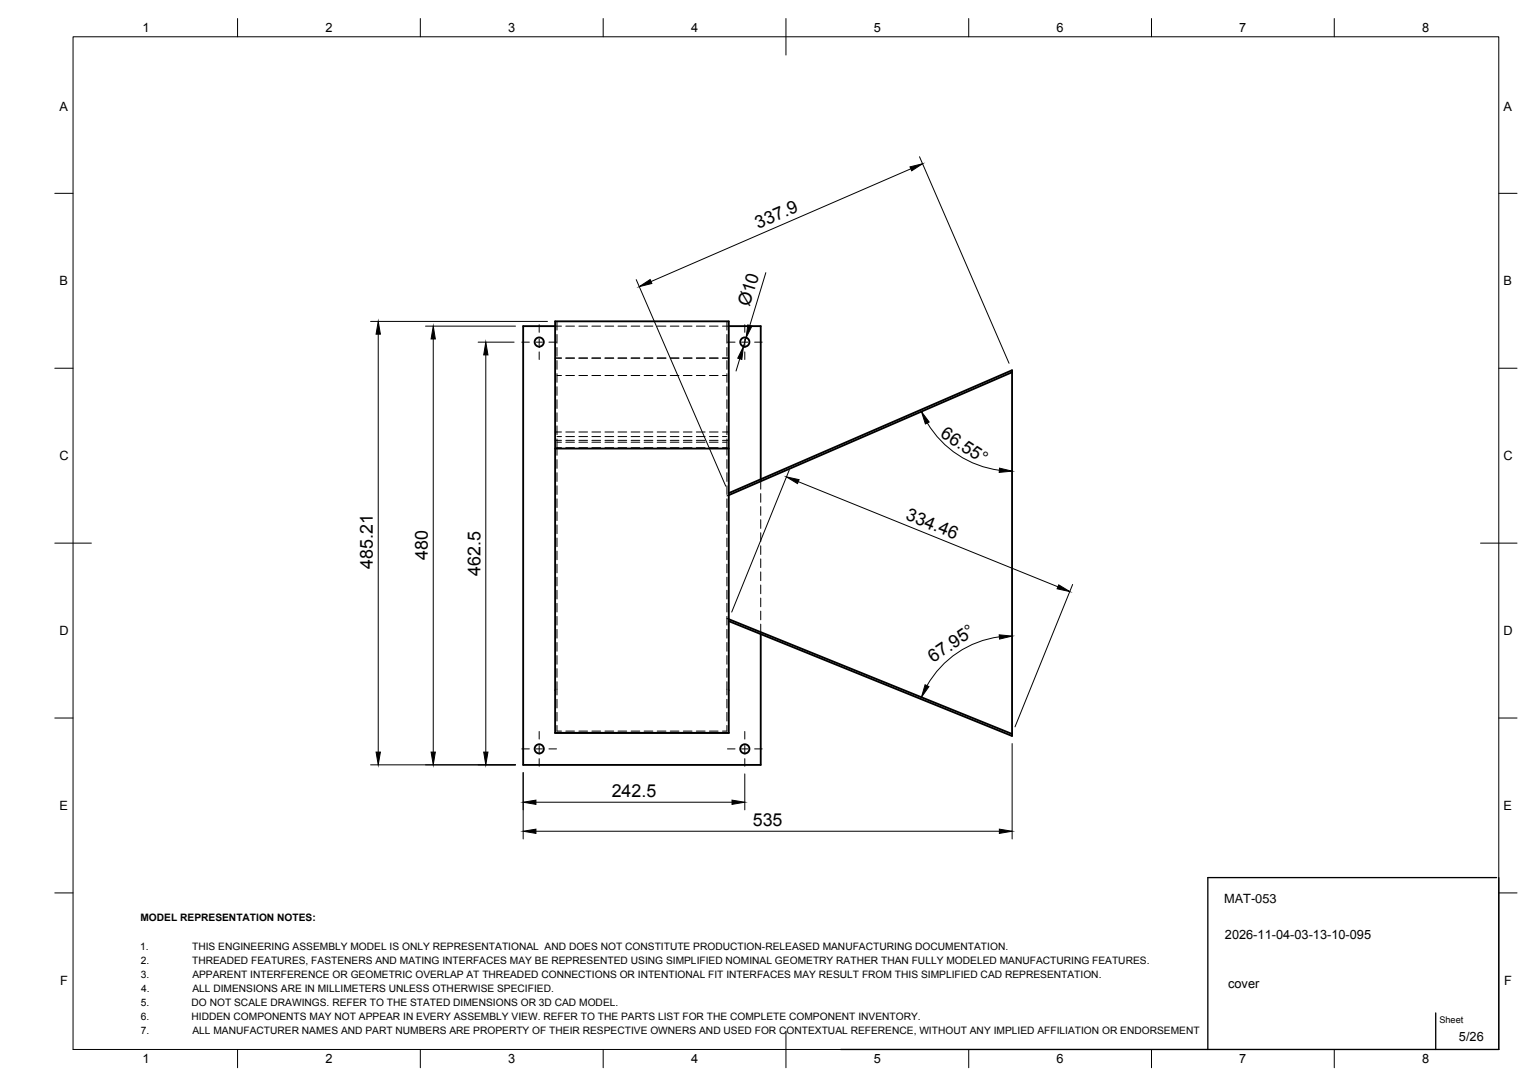
ISO-10303-21;
HEADER;
FILE_DESCRIPTION (('STEP AP214'),
    '1' );
FILE_NAME ('cover.step',
    '2026-10-10T03:43:58',
    ( '' ),
    ( '' ),
    'SwSTEP 2.0',
    'SolidWorks 2026',
    '' );
FILE_SCHEMA (( 'AUTOMOTIVE_DESIGN' ));
ENDSEC;

DATA;
#72=EDGE_CURVE ( 'NONE', #9244, #1149, #61881, .T. ) ;
#95=( NAMED_UNIT ( * ) SI_UNIT ( $, .STERADIAN. ) SOLID_ANGLE_UNIT ( ) );
#152=VECTOR ( 'NONE', #5107, 1000.000000000000000 ) ;
#372=ADVANCED_FACE ( 'NONE', ( #59703 ), #54424, .T. ) ;
#436=ORIENTED_EDGE ( 'NONE', *, *, #28005, .T. ) ;
#560=ORIENTED_EDGE ( 'NONE', *, *, #67855, .T. ) ;
#583=CARTESIAN_POINT ( 'NONE',  ( 544.6745185807129701, 190.0000000000000000, 34.73878747406611467 ) ) ;
#604=LINE ( 'NONE', #43156, #69293 ) ;
#627=EDGE_CURVE ( 'NONE', #45198, #50879, #47422, .T. ) ;
#655=CIRCLE ( 'NONE', #60208, 5.000000000000004441 ) ;
#687=LINE ( 'NONE', #32690, #59969 ) ;
#719=ORIENTED_EDGE ( 'NONE', *, *, #53021, .T. ) ;
#755=EDGE_LOOP ( 'NONE', ( #38002, #54803, #6340, #38216 ) ) ;
#761=AXIS2_PLACEMENT_3D ( 'NONE', #52678, #36171, #19998 ) ;
#765=CYLINDRICAL_SURFACE ( 'NONE', #45215, 498.0000000000000000 ) ;
#855=AXIS2_PLACEMENT_3D ( 'NONE', #17827, #11841, #44185 ) ;
#903=VECTOR ( 'NONE', #22935, 1000.000000000000227 ) ;
#955=ADVANCED_FACE ( 'NONE', ( #29059 ), #50502, .F. ) ;
#967=DIRECTION ( 'NONE',  ( 0.000000000000000000, -1.000000000000000000, 0.000000000000000000 ) ) ;
#1013=FACE_OUTER_BOUND ( 'NONE', #13752, .T. ) ;
#1016=EDGE_CURVE ( 'NONE', #28423, #15873, #49084, .T. ) ;
#1031=LINE ( 'NONE', #55528, #43434 ) ;
#1058=VECTOR ( 'NONE', #1739, 1000.000000000000000 ) ;
#1068=EDGE_LOOP ( 'NONE', ( #54688, #23963, #14484, #64716 ) ) ;
#1072=EDGE_LOOP ( 'NONE', ( #4972, #45772, #7897, #719 ) ) ;
#1100=EDGE_CURVE ( 'NONE', #68856, #49636, #25515, .T. ) ;
#1120=ORIENTED_EDGE ( 'NONE', *, *, #63162, .F. ) ;
#1139=DIRECTION ( 'NONE',  ( -0.000000000000000000, -1.000000000000000000, 0.000000000000000000 ) ) ;
#1149=VERTEX_POINT ( 'NONE', #58195 ) ;
#1267=CARTESIAN_POINT ( 'NONE',  ( 427.4999999999999432, 207.5000000000000284, 20.00000000000000000 ) ) ;
#1301=CARTESIAN_POINT ( 'NONE',  ( 329.1355598199468204, 190.0000000000000000, -129.5087625010780812 ) ) ;
#1353=ORIENTED_EDGE ( 'NONE', *, *, #66788, .F. ) ;
#1368=DIRECTION ( 'NONE',  ( 0.000000000000000000, 0.000000000000000000, -1.000000000000000000 ) ) ;
#1453=DIRECTION ( 'NONE',  ( -1.000000000000000000, -0.000000000000000000, -0.000000000000000000 ) ) ;
#1518=ORIENTED_EDGE ( 'NONE', *, *, #63162, .T. ) ;
#1528=FACE_OUTER_BOUND ( 'NONE', #26038, .T. ) ;
#1554=DIRECTION ( 'NONE',  ( 0.000000000000000000, -1.000000000000000000, 0.000000000000000000 ) ) ;
#1590=ADVANCED_FACE ( 'NONE', ( #39693 ), #61149, .F. ) ;
#1594=VERTEX_POINT ( 'NONE', #29141 ) ;
#1611=DIRECTION ( 'NONE',  ( 0.000000000000000000, 0.000000000000000000, -1.000000000000000000 ) ) ;
#1663=ADVANCED_FACE ( 'NONE', ( #69520, #10102 ), #63570, .F. ) ;
#1722=CARTESIAN_POINT ( 'NONE',  ( -17.50000000000000000, 207.5000000000000284, 0.000000000000000000 ) ) ;
#1724=LINE ( 'NONE', #12275, #14687 ) ;
#1739=DIRECTION ( 'NONE',  ( -1.000000000000000000, -0.000000000000000000, -0.000000000000000000 ) ) ;
#1850=EDGE_CURVE ( 'NONE', #58197, #53112, #45577, .T. ) ;
#1910=CARTESIAN_POINT ( 'NONE',  ( -3.306248862503413655, 500.0000000000000000, -51.64566090791306863 ) ) ;
#1921=PLANE ( 'NONE',  #11654 ) ;
#1944=AXIS2_PLACEMENT_3D ( 'NONE', #14779, #57012, #9163 ) ;
#2001=DIRECTION ( 'NONE',  ( -0.000000000000000000, 0.000000000000000000, 1.000000000000000000 ) ) ;
#2080=DIRECTION ( 'NONE',  ( -1.000000000000000000, 0.000000000000000000, 0.000000000000000000 ) ) ;
#2090=PLANE ( 'NONE',  #24134 ) ;
#2129=DIRECTION ( 'NONE',  ( 0.000000000000000000, 0.000000000000000000, -1.000000000000000000 ) ) ;
#2183=( GEOMETRIC_REPRESENTATION_CONTEXT ( 3 ) GLOBAL_UNCERTAINTY_ASSIGNED_CONTEXT ( ( #2954 ) ) GLOBAL_UNIT_ASSIGNED_CONTEXT ( ( #13188, #10650, #95 ) ) REPRESENTATION_CONTEXT ( 'NONE', 'WORKASPACE' ) );
#2294=VERTEX_POINT ( 'NONE', #16593 ) ;
#2340=CARTESIAN_POINT ( 'NONE',  ( 427.4999999999999432, -17.50000000000000000, 1.999999999999998224 ) ) ;
#2432=FACE_OUTER_BOUND ( 'NONE', #59132, .T. ) ;
#2454=FACE_OUTER_BOUND ( 'NONE', #34954, .T. ) ;
#2458=VECTOR ( 'NONE', #56262, 1000.000000000000000 ) ;
#2459=ORIENTED_EDGE ( 'NONE', *, *, #31851, .T. ) ;
#2461=CARTESIAN_POINT ( 'NONE',  ( -35.00000000000000000, -35.00000000000000000, 2.000000000000000000 ) ) ;
#2510=CARTESIAN_POINT ( 'NONE',  ( 432.4999999999999432, -17.50000000000000000, 1.999999999999998224 ) ) ;
#2542=EDGE_LOOP ( 'NONE', ( #55637, #55611, #67408, #62699 ) ) ;
#2549=CARTESIAN_POINT ( 'NONE',  ( -35.00000000000000000, 225.0000000000000000, 2.000000000000000000 ) ) ;
#2578=LINE ( 'NONE', #60620, #48950 ) ;
#2586=CARTESIAN_POINT ( 'NONE',  ( 124.4094311749753814, 190.0000000000000000, -91.28179539054374914 ) ) ;
#2597=CARTESIAN_POINT ( 'NONE',  ( 422.4999999999999432, -17.50000000000000000, 20.00000000000000000 ) ) ;
#2618=CARTESIAN_POINT ( 'NONE',  ( -12.50000000000000000, -17.50000000000000000, 1.999999999999998224 ) ) ;
#2633=DIRECTION ( 'NONE',  ( 0.000000000000000000, -0.000000000000000000, -1.000000000000000000 ) ) ;
#2634=EDGE_CURVE ( 'NONE', #39735, #19572, #687, .T. ) ;
#2720=LINE ( 'NONE', #3072, #17293 ) ;
#2774=CARTESIAN_POINT ( 'NONE',  ( 444.9999999999999432, 225.0000000000000000, 2.000000000000000000 ) ) ;
#2796=VECTOR ( 'NONE', #29277, 1000.000000000000000 ) ;
#2819=CARTESIAN_POINT ( 'NONE',  ( -35.00000000000000000, -35.00000000000000000, 2.000000000000000000 ) ) ;
#2900=DIRECTION ( 'NONE',  ( -0.000000000000000000, -0.000000000000000000, -1.000000000000000000 ) ) ;
#2931=ORIENTED_EDGE ( 'NONE', *, *, #21135, .T. ) ;
#2932=CARTESIAN_POINT ( 'NONE',  ( -17.50000000000000000, 207.5000000000000284, 20.00000000000000000 ) ) ;
#2954=UNCERTAINTY_MEASURE_WITH_UNIT (LENGTH_MEASURE( 1.000000000000000082E-05 ), #13188, 'distance_accuracy_value', 'NONE');
#2976=DIRECTION ( 'NONE',  ( 0.000000000000000000, -0.000000000000000000, -1.000000000000000000 ) ) ;
#3064=EDGE_CURVE ( 'NONE', #32859, #9244, #55362, .T. ) ;
#3069=EDGE_LOOP ( 'NONE', ( #53736, #43448 ) ) ;
#3072=CARTESIAN_POINT ( 'NONE',  ( -3.306248862503413655, 500.0000000000000000, -91.64566090791306863 ) ) ;
#3079=ORIENTED_EDGE ( 'NONE', *, *, #67167, .T. ) ;
#3080=ORIENTED_EDGE ( 'NONE', *, *, #68526, .T. ) ;
#3126=EDGE_LOOP ( 'NONE', ( #63304, #38150 ) ) ;
#3138=AXIS2_PLACEMENT_3D ( 'NONE', #31491, #3714, #68434 ) ;
#3199=CIRCLE ( 'NONE', #40248, 299.9999999999999432 ) ;
#3206=CARTESIAN_POINT ( 'NONE',  ( 262.2516123306975260, 190.0000000000000000, -21.28179539054375624 ) ) ;
#3323=ORIENTED_EDGE ( 'NONE', *, *, #68445, .F. ) ;
#3328=CARTESIAN_POINT ( 'NONE',  ( 46.68215785206009372, 190.0000000000000000, -77.29788463846088575 ) ) ;
#3448=ORIENTED_EDGE ( 'NONE', *, *, #37030, .T. ) ;
#3462=VERTEX_POINT ( 'NONE', #27498 ) ;
#3473=ORIENTED_EDGE ( 'NONE', *, *, #19374, .F. ) ;
#3528=ORIENTED_EDGE ( 'NONE', *, *, #31290, .F. ) ;
#3596=AXIS2_PLACEMENT_3D ( 'NONE', #19332, #9134, #56272 ) ;
#3663=EDGE_CURVE ( 'NONE', #23198, #50057, #6129, .T. ) ;
#3665=FACE_OUTER_BOUND ( 'NONE', #32196, .T. ) ;
#3714=DIRECTION ( 'NONE',  ( -0.000000000000000000, 0.000000000000000000, 1.000000000000000000 ) ) ;
#3749=CARTESIAN_POINT ( 'NONE',  ( 0.000000000000000000, 190.0000000000000000, 0.000000000000000000 ) ) ;
#3771=VECTOR ( 'NONE', #23467, 1000.000000000000000 ) ;
#3787=VECTOR ( 'NONE', #54739, 1000.000000000000000 ) ;
#3802=CARTESIAN_POINT ( 'NONE',  ( -17.50000000000000000, -17.50000000000000000, 20.00000000000000000 ) ) ;
#3835=ORIENTED_EDGE ( 'NONE', *, *, #21190, .F. ) ;
#3850=CARTESIAN_POINT ( 'NONE',  ( 99.71998884745383407, 0.000000000000000000, 7.478223336038896996 ) ) ;
#3887=DIRECTION ( 'NONE',  ( 0.000000000000000000, -0.000000000000000000, -1.000000000000000000 ) ) ;
#3923=ORIENTED_EDGE ( 'NONE', *, *, #39148, .F. ) ;
#3934=ORIENTED_EDGE ( 'NONE', *, *, #8106, .F. ) ;
#3972=LINE ( 'NONE', #57436, #13122 ) ;
#4135=DIRECTION ( 'NONE',  ( 0.000000000000000000, 1.000000000000000000, -0.000000000000000000 ) ) ;
#4164=DIRECTION ( 'NONE',  ( 0.000000000000000000, -0.000000000000000000, -1.000000000000000000 ) ) ;
#4185=CIRCLE ( 'NONE', #761, 89.99999999999997158 ) ;
#4233=EDGE_CURVE ( 'NONE', #6944, #45198, #13429, .T. ) ;
#4270=AXIS2_PLACEMENT_3D ( 'NONE', #11426, #20963, #48021 ) ;
#4274=EDGE_LOOP ( 'NONE', ( #32274, #55909, #20060, #69556 ) ) ;
#4399=CARTESIAN_POINT ( 'NONE',  ( 544.6745185807129701, 190.0000000000000000, 34.73878747406611467 ) ) ;
#4565=ORIENTED_EDGE ( 'NONE', *, *, #1100, .F. ) ;
#4656=LINE ( 'NONE', #52833, #38629 ) ;
#4697=DIRECTION ( 'NONE',  ( -0.000000000000000000, -0.000000000000000000, -1.000000000000000000 ) ) ;
#4773=ORIENTED_EDGE ( 'NONE', *, *, #26684, .T. ) ;
#4800=EDGE_LOOP ( 'NONE', ( #6610, #17998, #29657, #19956 ) ) ;
#4885=CIRCLE ( 'NONE', #59958, 500.0000000000000000 ) ;
#4916=DIRECTION ( 'NONE',  ( -1.000000000000000000, 0.000000000000000000, 0.000000000000000000 ) ) ;
#4972=ORIENTED_EDGE ( 'NONE', *, *, #28424, .T. ) ;
#4974=CARTESIAN_POINT ( 'NONE',  ( 432.4999999999999432, 207.5000000000000284, 20.00000000000000000 ) ) ;
#5079=AXIS2_PLACEMENT_3D ( 'NONE', #60400, #28035, #12215 ) ;
#5102=DIRECTION ( 'NONE',  ( -1.000000000000000000, 0.000000000000000000, 0.000000000000000000 ) ) ;
#5107=DIRECTION ( 'NONE',  ( 1.000000000000000000, 0.000000000000000000, 0.000000000000000000 ) ) ;
#5231=EDGE_LOOP ( 'NONE', ( #57842, #67743, #13618, #3448 ) ) ;
#5275=DIRECTION ( 'NONE',  ( 0.000000000000000000, 1.000000000000000000, -0.000000000000000000 ) ) ;
#5288=( LENGTH_UNIT ( ) NAMED_UNIT ( * ) SI_UNIT ( .MILLI., .METRE. ) );
#5353=DIRECTION ( 'NONE',  ( -0.000000000000000000, -0.000000000000000000, -1.000000000000000000 ) ) ;
#5418=CIRCLE ( 'NONE', #24575, 299.9999999999999432 ) ;
#5500=ORIENTED_EDGE ( 'NONE', *, *, #38822, .T. ) ;
#5510=DIRECTION ( 'NONE',  ( 0.000000000000000000, -0.000000000000000000, -1.000000000000000000 ) ) ;
#5607=EDGE_CURVE ( 'NONE', #68856, #56615, #2720, .T. ) ;
#5636=CARTESIAN_POINT ( 'NONE',  ( 450.2085304802404266, 0.000000000000000000, -250.0000000000000000 ) ) ;
#5692=PRODUCT_DEFINITION_CONTEXT ( 'detailed design', #47573, 'design' ) ;
#5753=ORIENTED_EDGE ( 'NONE', *, *, #24618, .F. ) ;
#5759=CARTESIAN_POINT ( 'NONE',  ( 311.8713128290285113, 2.000000000000001776, 346.5826552340383842 ) ) ;
#5841=DIRECTION ( 'NONE',  ( 1.000000000000000000, 0.000000000000000000, 0.000000000000000000 ) ) ;
#5867=DIRECTION ( 'NONE',  ( -0.3754025596372949636, 0.9268618657695261165, 0.000000000000000000 ) ) ;
#5916=CIRCLE ( 'NONE', #19450, 97.99999999999994316 ) ;
#5926=LINE ( 'NONE', #38296, #48690 ) ;
#5953=VERTEX_POINT ( 'NONE', #33957 ) ;
#5957=CYLINDRICAL_SURFACE ( 'NONE', #23378, 500.0000000000000000 ) ;
#6094=DIRECTION ( 'NONE',  ( -0.000000000000000000, 0.000000000000000000, -1.000000000000000000 ) ) ;
#6129=LINE ( 'NONE', #64891, #46370 ) ;
#6139=SHAPE_DEFINITION_REPRESENTATION ( #7501, #15003 ) ;
#6221=DIRECTION ( 'NONE',  ( -1.000000000000000000, 0.000000000000000000, 0.000000000000000000 ) ) ;
#6340=ORIENTED_EDGE ( 'NONE', *, *, #27885, .T. ) ;
#6385=CARTESIAN_POINT ( 'NONE',  ( 563.4809901518626702, 2.000000000000001776, 57.79371821540657095 ) ) ;
#6463=PLANE ( 'NONE',  #38849 ) ;
#6504=FACE_OUTER_BOUND ( 'NONE', #40019, .T. ) ;
#6610=ORIENTED_EDGE ( 'NONE', *, *, #41999, .T. ) ;
#6657=LINE ( 'NONE', #22839, #1058 ) ;
#6674=CARTESIAN_POINT ( 'NONE',  ( 410.0000000000000000, 190.0000000000000000, 2.000000000000000000 ) ) ;
#6707=CARTESIAN_POINT ( 'NONE',  ( 46.68215785206009372, 190.0000000000000000, -77.29788463846088575 ) ) ;
#6711=VERTEX_POINT ( 'NONE', #47309 ) ;
#6757=ADVANCED_FACE ( 'NONE', ( #38184 ), #17062, .F. ) ;
#6759=CARTESIAN_POINT ( 'NONE',  ( 563.4809901518626702, 188.0000000000000000, 57.79371821540657095 ) ) ;
#6779=PLANE ( 'NONE',  #31489 ) ;
#6842=CARTESIAN_POINT ( 'NONE',  ( 122.2516123306975402, 190.0000000000000000, -21.28179539054375624 ) ) ;
#6862=ORIENTED_EDGE ( 'NONE', *, *, #67221, .T. ) ;
#6869=CARTESIAN_POINT ( 'NONE',  ( -3.306248862503413655, 500.0000000000000000, -91.64566090791306863 ) ) ;
#6944=VERTEX_POINT ( 'NONE', #68400 ) ;
#6961=ORIENTED_EDGE ( 'NONE', *, *, #32632, .F. ) ;
#7063=DIRECTION ( 'NONE',  ( 0.000000000000000000, 0.000000000000000000, 1.000000000000000000 ) ) ;
#7291=ORIENTED_EDGE ( 'NONE', *, *, #27232, .F. ) ;
#7305=AXIS2_PLACEMENT_3D ( 'NONE', #42807, #17110, #5867 ) ;
#7363=FACE_BOUND ( 'NONE', #15953, .T. ) ;
#7407=EDGE_CURVE ( 'NONE', #8775, #26863, #45567, .T. ) ;
#7420=LINE ( 'NONE', #8453, #39043 ) ;
#7477=PLANE ( 'NONE',  #30552 ) ;
#7487=ORIENTED_EDGE ( 'NONE', *, *, #33804, .T. ) ;
#7501=PRODUCT_DEFINITION_SHAPE ( 'NONE', 'NONE',  #58101 ) ;
#7566=CARTESIAN_POINT ( 'NONE',  ( -17.50000000000000000, -17.50000000000000000, 0.000000000000000000 ) ) ;
#7586=ORIENTED_EDGE ( 'NONE', *, *, #16733, .T. ) ;
#7611=VECTOR ( 'NONE', #14241, 1000.000000000000000 ) ;
#7799=EDGE_CURVE ( 'NONE', #3462, #61751, #2578, .T. ) ;
#7834=AXIS2_PLACEMENT_3D ( 'NONE', #47808, #36233, #21092 ) ;
#7881=ADVANCED_FACE ( 'NONE', ( #1528 ), #6463, .F. ) ;
#7897=ORIENTED_EDGE ( 'NONE', *, *, #23089, .F. ) ;
#7903=DIRECTION ( 'NONE',  ( 0.000000000000000000, 0.000000000000000000, -1.000000000000000000 ) ) ;
#7931=DIRECTION ( 'NONE',  ( -1.000000000000000000, 0.000000000000000000, -0.000000000000000000 ) ) ;
#7940=DIRECTION ( 'NONE',  ( -0.000000000000000000, 0.000000000000000000, 1.000000000000000000 ) ) ;
#7942=ORIENTED_EDGE ( 'NONE', *, *, #68285, .T. ) ;
#7968=LINE ( 'NONE', #18180, #3771 ) ;
#8106=EDGE_CURVE ( 'NONE', #22374, #22712, #21502, .T. ) ;
#8207=VERTEX_POINT ( 'NONE', #25694 ) ;
#8224=DIRECTION ( 'NONE',  ( -0.000000000000000000, -0.000000000000000000, -1.000000000000000000 ) ) ;
#8319=DIRECTION ( 'NONE',  ( 1.000000000000000000, 0.000000000000000000, 0.000000000000000000 ) ) ;
#8380=DIRECTION ( 'NONE',  ( 0.000000000000000000, 0.000000000000000000, -1.000000000000000000 ) ) ;
#8381=CARTESIAN_POINT ( 'NONE',  ( 0.000000000000000000, 190.0000000000000000, 2.000000000000000000 ) ) ;
#8450=AXIS2_PLACEMENT_3D ( 'NONE', #33478, #67813, #23266 ) ;
#8453=CARTESIAN_POINT ( 'NONE',  ( 149.5059104800819796, -64.94516058774519252, -90.98255102680806772 ) ) ;
#8775=VERTEX_POINT ( 'NONE', #2510 ) ;
#8863=VERTEX_POINT ( 'NONE', #23623 ) ;
#8943=SURFACE_STYLE_FILL_AREA ( #57135 ) ;
#9097=EDGE_CURVE ( 'NONE', #27270, #54323, #13093, .T. ) ;
#9121=ORIENTED_EDGE ( 'NONE', *, *, #21343, .F. ) ;
#9134=DIRECTION ( 'NONE',  ( -0.000000000000000000, -1.000000000000000000, 0.000000000000000000 ) ) ;
#9138=EDGE_CURVE ( 'NONE', #33323, #38900, #1031, .T. ) ;
#9163=DIRECTION ( 'NONE',  ( 0.000000000000000000, 0.000000000000000000, -1.000000000000000000 ) ) ;
#9244=VERTEX_POINT ( 'NONE', #2819 ) ;
#9273=AXIS2_PLACEMENT_3D ( 'NONE', #41737, #38090, #32823 ) ;
#9341=FACE_BOUND ( 'NONE', #3126, .T. ) ;
#9414=DIRECTION ( 'NONE',  ( 0.000000000000000000, -1.000000000000000000, 0.000000000000000000 ) ) ;
#9440=FACE_OUTER_BOUND ( 'NONE', #1072, .T. ) ;
#9612=VECTOR ( 'NONE', #27215, 1000.000000000000000 ) ;
#9657=VECTOR ( 'NONE', #33393, 1000.000000000000000 ) ;
#9977=ORIENTED_EDGE ( 'NONE', *, *, #39148, .T. ) ;
#10020=CARTESIAN_POINT ( 'NONE',  ( 410.0000000000000000, 0.000000000000000000, 2.000000000000000000 ) ) ;
#10102=FACE_OUTER_BOUND ( 'NONE', #57610, .T. ) ;
#10125=ORIENTED_EDGE ( 'NONE', *, *, #16907, .T. ) ;
#10159=ORIENTED_EDGE ( 'NONE', *, *, #48623, .F. ) ;
#10170=EDGE_CURVE ( 'NONE', #54229, #41559, #67130, .T. ) ;
#10249=CARTESIAN_POINT ( 'NONE',  ( 262.2516123306975260, 190.0000000000000000, -91.28179539054376335 ) ) ;
#10275=ORIENTED_EDGE ( 'NONE', *, *, #10170, .F. ) ;
#10410=CARTESIAN_POINT ( 'NONE',  ( 0.000000000000000000, -0.2591992991291388049, -2.646296226153046938 ) ) ;
#10519=ORIENTED_EDGE ( 'NONE', *, *, #68285, .F. ) ;
#10650=( NAMED_UNIT ( * ) PLANE_ANGLE_UNIT ( ) SI_UNIT ( $, .RADIAN. ) );
#10773=ORIENTED_EDGE ( 'NONE', *, *, #29862, .T. ) ;
#10921=EDGE_CURVE ( 'NONE', #15873, #38606, #31220, .T. ) ;
#10954=ORIENTED_EDGE ( 'NONE', *, *, #41139, .T. ) ;
#10965=DIRECTION ( 'NONE',  ( 0.000000000000000000, 0.000000000000000000, -1.000000000000000000 ) ) ;
#11077=ORIENTED_EDGE ( 'NONE', *, *, #13353, .T. ) ;
#11182=EDGE_CURVE ( 'NONE', #44112, #5953, #40299, .T. ) ;
#11317=EDGE_CURVE ( 'NONE', #53112, #14479, #18751, .T. ) ;
#11426=CARTESIAN_POINT ( 'NONE',  ( -17.50000000000000000, 207.5000000000000284, 1.999999999999998224 ) ) ;
#11442=ORIENTED_EDGE ( 'NONE', *, *, #63589, .T. ) ;
#11449=( GEOMETRIC_REPRESENTATION_CONTEXT ( 3 ) GLOBAL_UNCERTAINTY_ASSIGNED_CONTEXT ( ( #14872 ) ) GLOBAL_UNIT_ASSIGNED_CONTEXT ( ( #5288, #42902, #58396 ) ) REPRESENTATION_CONTEXT ( 'NONE', 'WORKASPACE' ) );
#11522=CARTESIAN_POINT ( 'NONE',  ( -35.00000000000000000, 225.0000000000000000, 2.000000000000000000 ) ) ;
#11524=EDGE_LOOP ( 'NONE', ( #31151, #7487, #34608, #36208 ) ) ;
#11548=EDGE_CURVE ( 'NONE', #5953, #28478, #3199, .T. ) ;
#11580=VERTEX_POINT ( 'NONE', #21515 ) ;
#11643=VECTOR ( 'NONE', #49675, 1000.000000000000000 ) ;
#11652=DIRECTION ( 'NONE',  ( -0.000000000000000000, -1.000000000000000000, -0.000000000000000000 ) ) ;
#11654=AXIS2_PLACEMENT_3D ( 'NONE', #23374, #44819, #33227 ) ;
#11701=CARTESIAN_POINT ( 'NONE',  ( -35.00000000000000000, 225.0000000000000000, 0.000000000000000000 ) ) ;
#11723=ADVANCED_FACE ( 'NONE', ( #40139 ), #19024, .T. ) ;
#11747=FACE_OUTER_BOUND ( 'NONE', #2542, .T. ) ;
#11770=DIRECTION ( 'NONE',  ( -0.000000000000000000, -1.000000000000000000, -0.000000000000000000 ) ) ;
#11789=ORIENTED_EDGE ( 'NONE', *, *, #4233, .T. ) ;
#11799=ADVANCED_FACE ( 'NONE', ( #22913, #60890 ), #52419, .T. ) ;
#11813=AXIS2_PLACEMENT_3D ( 'NONE', #29215, #42438, #18665 ) ;
#11841=DIRECTION ( 'NONE',  ( 0.000000000000000000, 1.000000000000000000, 0.000000000000000000 ) ) ;
#11878=CARTESIAN_POINT ( 'NONE',  ( 410.0000000000000000, 0.000000000000000000, 2.000000000000000000 ) ) ;
#11926=ADVANCED_FACE ( 'NONE', ( #51728 ), #36243, .F. ) ;
#11952=VERTEX_POINT ( 'NONE', #36593 ) ;
#12022=ORIENTED_EDGE ( 'NONE', *, *, #68445, .T. ) ;
#12032=LINE ( 'NONE', #39126, #903 ) ;
#12055=CARTESIAN_POINT ( 'NONE',  ( 410.0000000000000000, 0.000000000000000000, -90.00000000000000000 ) ) ;
#12148=EDGE_LOOP ( 'NONE', ( #3835, #10275 ) ) ;
#12193=ORIENTED_EDGE ( 'NONE', *, *, #16765, .F. ) ;
#12196=DIRECTION ( 'NONE',  ( 1.000000000000000000, 0.000000000000000000, 0.000000000000000000 ) ) ;
#12203=PLANE ( 'NONE',  #14036 ) ;
#12215=DIRECTION ( 'NONE',  ( 0.000000000000000000, 0.000000000000000000, -1.000000000000000000 ) ) ;
#12275=CARTESIAN_POINT ( 'NONE',  ( 329.1355598199468204, 190.0000000000000000, -129.5087625010780812 ) ) ;
#12361=CARTESIAN_POINT ( 'NONE',  ( 0.000000000000000000, 0.000000000000000000, 2.000000000000000000 ) ) ;
#12363=VECTOR ( 'NONE', #69040, 999.9999999999998863 ) ;
#12429=AXIS2_PLACEMENT_3D ( 'NONE', #47040, #29826, #41426 ) ;
#12549=CARTESIAN_POINT ( 'NONE',  ( 410.0000000000000000, 0.000000000000000000, 0.000000000000000000 ) ) ;
#12624=LINE ( 'NONE', #23874, #55752 ) ;
#12713=EDGE_CURVE ( 'NONE', #22712, #49636, #17250, .T. ) ;
#12777=ORIENTED_EDGE ( 'NONE', *, *, #32544, .F. ) ;
#12905=EDGE_CURVE ( 'NONE', #52426, #26511, #7420, .T. ) ;
#12972=CARTESIAN_POINT ( 'NONE',  ( 563.4809901518626702, 190.0000000000000000, 57.79371821540657095 ) ) ;
#12999=DIRECTION ( 'NONE',  ( 0.000000000000000000, 0.000000000000000000, -1.000000000000000000 ) ) ;
#13016=LINE ( 'NONE', #49929, #20048 ) ;
#13093=CIRCLE ( 'NONE', #20960, 5.000000000000000888 ) ;
#13102=ORIENTED_EDGE ( 'NONE', *, *, #35948, .T. ) ;
#13103=CARTESIAN_POINT ( 'NONE',  ( 311.0133388548732114, 190.0000000000000000, -153.4166086460792826 ) ) ;
#13122=VECTOR ( 'NONE', #19804, 1000.000000000000000 ) ;
#13125=EDGE_CURVE ( 'NONE', #28478, #3462, #24663, .T. ) ;
#13168=EDGE_CURVE ( 'NONE', #34560, #66549, #57932, .T. ) ;
#13183=DIRECTION ( 'NONE',  ( 0.000000000000000000, 0.000000000000000000, -1.000000000000000000 ) ) ;
#13184=DIRECTION ( 'NONE',  ( -0.000000000000000000, -1.000000000000000000, -0.000000000000000000 ) ) ;
#13188=( LENGTH_UNIT ( ) NAMED_UNIT ( * ) SI_UNIT ( .MILLI., .METRE. ) );
#13223=DIRECTION ( 'NONE',  ( 0.000000000000000000, 1.000000000000000000, -0.000000000000000000 ) ) ;
#13245=CARTESIAN_POINT ( 'NONE',  ( 46.68215785206009372, 0.000000000000000000, -77.29788463846088575 ) ) ;
#13340=CARTESIAN_POINT ( 'NONE',  ( 563.4809901518626702, 190.0000000000000000, 57.79371821540657095 ) ) ;
#13353=EDGE_CURVE ( 'NONE', #8863, #25048, #62814, .T. ) ;
#13429=LINE ( 'NONE', #21129, #25103 ) ;
#13468=ORIENTED_EDGE ( 'NONE', *, *, #51660, .T. ) ;
#13476=DIRECTION ( 'NONE',  ( -0.000000000000000000, 0.000000000000000000, 1.000000000000000000 ) ) ;
#13526=CARTESIAN_POINT ( 'NONE',  ( 563.4809901518626702, 190.0000000000000000, 57.79371821540657095 ) ) ;
#13618=ORIENTED_EDGE ( 'NONE', *, *, #45185, .F. ) ;
#13665=ADVANCED_FACE ( 'NONE', ( #57691 ), #14768, .T. ) ;
#13674=CARTESIAN_POINT ( 'NONE',  ( 432.4999999999999432, 207.5000000000000284, 0.000000000000000000 ) ) ;
#13752=EDGE_LOOP ( 'NONE', ( #53113, #24876, #68609, #43593 ) ) ;
#13763=DIRECTION ( 'NONE',  ( -1.000000000000000000, 0.000000000000000000, 0.000000000000000000 ) ) ;
#13773=VECTOR ( 'NONE', #44763, 1000.000000000000000 ) ;
#13804=ORIENTED_EDGE ( 'NONE', *, *, #27232, .T. ) ;
#13820=ADVANCED_FACE ( 'NONE', ( #1013 ), #22114, .T. ) ;
#14009=FACE_OUTER_BOUND ( 'NONE', #755, .T. ) ;
#14021=LINE ( 'NONE', #28823, #23274 ) ;
#14036=AXIS2_PLACEMENT_3D ( 'NONE', #50870, #38944, #49464 ) ;
#14064=CIRCLE ( 'NONE', #8450, 91.99999999999997158 ) ;
#14066=DIRECTION ( 'NONE',  ( -1.000000000000000000, 0.000000000000000000, 0.000000000000000000 ) ) ;
#14069=ADVANCED_FACE ( 'NONE', ( #21338 ), #48744, .T. ) ;
#14074=VECTOR ( 'NONE', #20124, 1000.000000000000000 ) ;
#14241=DIRECTION ( 'NONE',  ( -0.000000000000000000, -0.000000000000000000, -1.000000000000000000 ) ) ;
#14283=PLANE ( 'NONE',  #3138 ) ;
#14349=CARTESIAN_POINT ( 'NONE',  ( -35.00000000000000000, 225.0000000000000000, 2.000000000000000000 ) ) ;
#14368=ORIENTED_EDGE ( 'NONE', *, *, #10921, .T. ) ;
#14392=ORIENTED_EDGE ( 'NONE', *, *, #32938, .T. ) ;
#14449=VERTEX_POINT ( 'NONE', #42029 ) ;
#14479=VERTEX_POINT ( 'NONE', #21949 ) ;
#14484=ORIENTED_EDGE ( 'NONE', *, *, #57557, .T. ) ;
#14687=VECTOR ( 'NONE', #35115, 1000.000000000000000 ) ;
#14706=LINE ( 'NONE', #2774, #68755 ) ;
#14749=VERTEX_POINT ( 'NONE', #18770 ) ;
#14768=PLANE ( 'NONE',  #7834 ) ;
#14779=CARTESIAN_POINT ( 'NONE',  ( 99.71998884745383407, 190.0000000000000000, 7.478223336038896996 ) ) ;
#14858=CARTESIAN_POINT ( 'NONE',  ( 0.000000000000000000, 190.0000000000000000, 2.000000000000000000 ) ) ;
#14872=UNCERTAINTY_MEASURE_WITH_UNIT (LENGTH_MEASURE( 1.000000000000000082E-05 ), #5288, 'distance_accuracy_value', 'NONE');
#14898=ORIENTED_EDGE ( 'NONE', *, *, #58658, .F. ) ;
#14899=ORIENTED_EDGE ( 'NONE', *, *, #67508, .F. ) ;
#15003=SHAPE_REPRESENTATION ( 'cover', ( #66832 ), #17430 ) ;
#15021=ORIENTED_EDGE ( 'NONE', *, *, #7407, .T. ) ;
#15238=CARTESIAN_POINT ( 'NONE',  ( 0.000000000000000000, 0.000000000000000000, 2.000000000000000000 ) ) ;
#15394=DIRECTION ( 'NONE',  ( -0.000000000000000000, -0.000000000000000000, -1.000000000000000000 ) ) ;
#15437=AXIS2_PLACEMENT_3D ( 'NONE', #3850, #41133, #46749 ) ;
#15622=VERTEX_POINT ( 'NONE', #38819 ) ;
#15827=FACE_OUTER_BOUND ( 'NONE', #27928, .T. ) ;
#15828=LINE ( 'NONE', #58723, #40646 ) ;
#15837=AXIS2_PLACEMENT_3D ( 'NONE', #19221, #50895, #46998 ) ;
#15865=DIRECTION ( 'NONE',  ( -0.000000000000000000, -0.000000000000000000, -1.000000000000000000 ) ) ;
#15873=VERTEX_POINT ( 'NONE', #42942 ) ;
#15876=LINE ( 'NONE', #4974, #14074 ) ;
#15953=EDGE_LOOP ( 'NONE', ( #28406, #25946, #47626, #2459 ) ) ;
#15967=DIRECTION ( 'NONE',  ( 1.000000000000000000, 0.000000000000000000, -0.000000000000000000 ) ) ;
#16058=DIRECTION ( 'NONE',  ( 1.000000000000000000, 0.000000000000000000, 0.000000000000000000 ) ) ;
#16153=DIRECTION ( 'NONE',  ( -1.000000000000000000, -0.000000000000000000, -0.000000000000000000 ) ) ;
#16229=CARTESIAN_POINT ( 'NONE',  ( 125.2194818923508848, 188.0000000000000000, 7.478223336038896996 ) ) ;
#16312=CARTESIAN_POINT ( 'NONE',  ( 0.000000000000000000, 190.0000000000000000, 2.000000000000000000 ) ) ;
#16334=ORIENTED_EDGE ( 'NONE', *, *, #21343, .T. ) ;
#16348=CARTESIAN_POINT ( 'NONE',  ( -17.50000000000000000, 207.5000000000000284, 1.999999999999998224 ) ) ;
#16361=VERTEX_POINT ( 'NONE', #2586 ) ;
#16510=FACE_OUTER_BOUND ( 'NONE', #25888, .T. ) ;
#16593=CARTESIAN_POINT ( 'NONE',  ( 432.4999999999999432, -17.50000000000000000, 0.000000000000000000 ) ) ;
#16598=EDGE_CURVE ( 'NONE', #43800, #24193, #60889, .T. ) ;
#16604=CIRCLE ( 'NONE', #4270, 5.000000000000000888 ) ;
#16652=LINE ( 'NONE', #53237, #64671 ) ;
#16733=EDGE_CURVE ( 'NONE', #23556, #19234, #26033, .T. ) ;
#16740=DIRECTION ( 'NONE',  ( -1.000000000000000000, 0.000000000000000000, 0.000000000000000000 ) ) ;
#16752=DIRECTION ( 'NONE',  ( 0.000000000000000000, 0.000000000000000000, -1.000000000000000000 ) ) ;
#16765=EDGE_CURVE ( 'NONE', #52426, #16361, #42872, .T. ) ;
#16805=VECTOR ( 'NONE', #68316, 1000.000000000000000 ) ;
#16870=FILL_AREA_STYLE ('',( #69571 ) ) ;
#16873=ORIENTED_EDGE ( 'NONE', *, *, #19374, .T. ) ;
#16902=EDGE_CURVE ( 'NONE', #18178, #27607, #49897, .T. ) ;
#16907=EDGE_CURVE ( 'NONE', #17378, #28478, #1724, .T. ) ;
#16929=AXIS2_PLACEMENT_3D ( 'NONE', #24746, #55704, #56055 ) ;
#16954=CARTESIAN_POINT ( 'NONE',  ( 311.8713128290285113, 190.0000000000000000, 346.5826552340383842 ) ) ;
#16971=EDGE_LOOP ( 'NONE', ( #34913, #19927, #24153, #42529 ) ) ;
#16994=PLANE ( 'NONE',  #43317 ) ;
#17021=DIRECTION ( 'NONE',  ( -0.000000000000000000, -1.000000000000000000, -0.000000000000000000 ) ) ;
#17062=PLANE ( 'NONE',  #64592 ) ;
#17067=ADVANCED_FACE ( 'NONE', ( #52332 ), #62894, .F. ) ;
#17100=CARTESIAN_POINT ( 'NONE',  ( 329.1355598199467636, 2.000000000000001776, -129.5087625010780812 ) ) ;
#17110=DIRECTION ( 'NONE',  ( 0.9268618657695262275, 0.3754025596372950191, 0.000000000000000000 ) ) ;
#17173=DIRECTION ( 'NONE',  ( 0.000000000000000000, 0.000000000000000000, -1.000000000000000000 ) ) ;
#17206=DIRECTION ( 'NONE',  ( -0.000000000000000000, -1.000000000000000000, -0.000000000000000000 ) ) ;
#17226=CIRCLE ( 'NONE', #65550, 5.000000000000004441 ) ;
#17231=VECTOR ( 'NONE', #54501, 1000.000000000000000 ) ;
#17233=VERTEX_POINT ( 'NONE', #69192 ) ;
#17250=LINE ( 'NONE', #49250, #63738 ) ;
#17293=VECTOR ( 'NONE', #19939, 1000.000000000000000 ) ;
#17327=LINE ( 'NONE', #11701, #11643 ) ;
#17378=VERTEX_POINT ( 'NONE', #61337 ) ;
#17430=( GEOMETRIC_REPRESENTATION_CONTEXT ( 3 ) GLOBAL_UNCERTAINTY_ASSIGNED_CONTEXT ( ( #29000 ) ) GLOBAL_UNIT_ASSIGNED_CONTEXT ( ( #46628, #56851, #51226 ) ) REPRESENTATION_CONTEXT ( 'NONE', 'WORKASPACE' ) );
#17593=PRODUCT_DEFINITION_FORMATION_WITH_SPECIFIED_SOURCE ( 'ANY', '', #45109, .NOT_KNOWN. ) ;
#17597=ORIENTED_EDGE ( 'NONE', *, *, #58189, .F. ) ;
#17667=EDGE_CURVE ( 'NONE', #28478, #25024, #15828, .T. ) ;
#17671=DIRECTION ( 'NONE',  ( -0.000000000000000000, 0.001173758924898823768, 0.9999993111447559313 ) ) ;
#17672=DIRECTION ( 'NONE',  ( 0.000000000000000000, 1.000000000000000000, -0.000000000000000000 ) ) ;
#17688=ORIENTED_EDGE ( 'NONE', *, *, #16902, .F. ) ;
#17708=ORIENTED_EDGE ( 'NONE', *, *, #68531, .F. ) ;
#17737=ORIENTED_EDGE ( 'NONE', *, *, #49048, .F. ) ;
#17747=ORIENTED_EDGE ( 'NONE', *, *, #33006, .F. ) ;
#17827=CARTESIAN_POINT ( 'NONE',  ( -35.00000000000000000, -35.00000000000000000, 2.000000000000000000 ) ) ;
#17870=CARTESIAN_POINT ( 'NONE',  ( 0.000000000000000000, 0.000000000000000000, 2.000000000000000000 ) ) ;
#17933=DIRECTION ( 'NONE',  ( 0.000000000000000000, 0.000000000000000000, -1.000000000000000000 ) ) ;
#17970=ORIENTED_EDGE ( 'NONE', *, *, #59862, .T. ) ;
#17998=ORIENTED_EDGE ( 'NONE', *, *, #72, .F. ) ;
#17999=DIRECTION ( 'NONE',  ( 0.000000000000000000, -0.000000000000000000, -1.000000000000000000 ) ) ;
#18036=MANIFOLD_SOLID_BREP ( 'Cut-Extrude1', #38393 ) ;
#18039=DIRECTION ( 'NONE',  ( 0.000000000000000000, -0.000000000000000000, -1.000000000000000000 ) ) ;
#18053=VECTOR ( 'NONE', #53939, 1000.000000000000000 ) ;
#18147=DIRECTION ( 'NONE',  ( -0.000000000000000000, -0.000000000000000000, -1.000000000000000000 ) ) ;
#18165=VECTOR ( 'NONE', #53831, 1000.000000000000000 ) ;
#18178=VERTEX_POINT ( 'NONE', #6674 ) ;
#18180=CARTESIAN_POINT ( 'NONE',  ( -12.50000000000000000, -17.50000000000000000, 20.00000000000000000 ) ) ;
#18281=CARTESIAN_POINT ( 'NONE',  ( -1.148430018225573557, 500.0000000000000000, -53.65523180892861177 ) ) ;
#18330=PLANE ( 'NONE',  #31153 ) ;
#18365=CARTESIAN_POINT ( 'NONE',  ( 450.2085304802404835, 0.000000000000000000, -219.9999999999999147 ) ) ;
#18402=AXIS2_PLACEMENT_3D ( 'NONE', #59592, #11770, #22328 ) ;
#18447=VECTOR ( 'NONE', #8224, 1000.000000000000000 ) ;
#18452=DIRECTION ( 'NONE',  ( -0.000000000000000000, -1.000000000000000000, 0.000000000000000000 ) ) ;
#18494=ORIENTED_EDGE ( 'NONE', *, *, #43804, .T. ) ;
#18520=ADVANCED_FACE ( 'NONE', ( #62496 ), #67427, .F. ) ;
#18593=DIRECTION ( 'NONE',  ( 0.000000000000000000, 1.000000000000000000, 0.000000000000000000 ) ) ;
#18595=AXIS2_PLACEMENT_3D ( 'NONE', #1722, #28448, #48480 ) ;
#18603=CARTESIAN_POINT ( 'NONE',  ( 0.000000000000000000, 190.0000000000000000, 0.000000000000000000 ) ) ;
#18611=CARTESIAN_POINT ( 'NONE',  ( 0.000000000000000000, 190.0000000000000000, 0.000000000000000000 ) ) ;
#18665=DIRECTION ( 'NONE',  ( 1.000000000000000000, 0.000000000000000000, 0.000000000000000000 ) ) ;
#18750=EDGE_CURVE ( 'NONE', #66549, #23198, #39287, .T. ) ;
#18751=CIRCLE ( 'NONE', #34643, 498.0000000000000000 ) ;
#18770=CARTESIAN_POINT ( 'NONE',  ( 444.9999999999999432, -35.00000000000000000, 2.000000000000000000 ) ) ;
#18944=CIRCLE ( 'NONE', #34720, 5.000000000000004441 ) ;
#18973=LINE ( 'NONE', #40422, #35773 ) ;
#18984=DIRECTION ( 'NONE',  ( -0.000000000000000000, -0.000000000000000000, -1.000000000000000000 ) ) ;
#19000=CYLINDRICAL_SURFACE ( 'NONE', #43736, 5.000000000000000888 ) ;
#19024=PLANE ( 'NONE',  #41354 ) ;
#19066=LINE ( 'NONE', #40520, #63922 ) ;
#19072=AXIS2_PLACEMENT_3D ( 'NONE', #583, #43823, #16752 ) ;
#19158=ORIENTED_EDGE ( 'NONE', *, *, #29375, .F. ) ;
#19221=CARTESIAN_POINT ( 'NONE',  ( 311.8713128290285113, 190.0000000000000000, 346.5826552340383842 ) ) ;
#19234=VERTEX_POINT ( 'NONE', #5636 ) ;
#19254=DIRECTION ( 'NONE',  ( 0.000000000000000000, 0.000000000000000000, -1.000000000000000000 ) ) ;
#19327=LINE ( 'NONE', #23917, #25538 ) ;
#19332=CARTESIAN_POINT ( 'NONE',  ( 563.4809901518626702, 188.0000000000000000, 57.79371821540657095 ) ) ;
#19374=EDGE_CURVE ( 'NONE', #17233, #11580, #36457, .T. ) ;
#19450=AXIS2_PLACEMENT_3D ( 'NONE', #30179, #4135, #8380 ) ;
#19572=VERTEX_POINT ( 'NONE', #43444 ) ;
#19598=AXIS2_PLACEMENT_3D ( 'NONE', #16348, #33238, #37113 ) ;
#19601=AXIS2_PLACEMENT_3D ( 'NONE', #43581, #32353, #37613 ) ;
#19642=LINE ( 'NONE', #18611, #34530 ) ;
#19792=ORIENTED_EDGE ( 'NONE', *, *, #11548, .T. ) ;
#19799=DIRECTION ( 'NONE',  ( -0.000000000000000000, -0.000000000000000000, -1.000000000000000000 ) ) ;
#19804=DIRECTION ( 'NONE',  ( 0.000000000000000000, 0.000000000000000000, -1.000000000000000000 ) ) ;
#19815=EDGE_LOOP ( 'NONE', ( #26290, #49775, #10519, #19869 ) ) ;
#19840=SURFACE_STYLE_USAGE ( .BOTH. , #68040 ) ;
#19846=CARTESIAN_POINT ( 'NONE',  ( 444.9999999999999432, 225.0000000000000000, 0.000000000000000000 ) ) ;
#19852=DIRECTION ( 'NONE',  ( -1.000000000000000000, 0.000000000000000000, 0.000000000000000000 ) ) ;
#19859=ADVANCED_FACE ( 'NONE', ( #44903 ), #12203, .T. ) ;
#19869=ORIENTED_EDGE ( 'NONE', *, *, #62745, .T. ) ;
#19927=ORIENTED_EDGE ( 'NONE', *, *, #48623, .T. ) ;
#19939=DIRECTION ( 'NONE',  ( -1.000000000000000000, -0.000000000000000000, -0.000000000000000000 ) ) ;
#19956=ORIENTED_EDGE ( 'NONE', *, *, #50653, .T. ) ;
#19960=EDGE_LOOP ( 'NONE', ( #16873, #20474, #9121, #42355 ) ) ;
#19998=DIRECTION ( 'NONE',  ( 0.000000000000000000, 0.000000000000000000, -1.000000000000000000 ) ) ;
#20048=VECTOR ( 'NONE', #17933, 1000.000000000000000 ) ;
#20060=ORIENTED_EDGE ( 'NONE', *, *, #25029, .F. ) ;
#20124=DIRECTION ( 'NONE',  ( -0.000000000000000000, -0.000000000000000000, -1.000000000000000000 ) ) ;
#20293=DIRECTION ( 'NONE',  ( -0.000000000000000000, -1.000000000000000000, 0.000000000000000000 ) ) ;
#20317=CARTESIAN_POINT ( 'NONE',  ( 410.0000000000000000, 190.0000000000000000, 0.000000000000000000 ) ) ;
#20463=LINE ( 'NONE', #35272, #46748 ) ;
#20474=ORIENTED_EDGE ( 'NONE', *, *, #36518, .F. ) ;
#20579=FACE_BOUND ( 'NONE', #51834, .T. ) ;
#20644=ADVANCED_FACE ( 'NONE', ( #45390 ), #45743, .F. ) ;
#20732=ORIENTED_EDGE ( 'NONE', *, *, #34405, .T. ) ;
#20840=VECTOR ( 'NONE', #45212, 1000.000000000000000 ) ;
#20960=AXIS2_PLACEMENT_3D ( 'NONE', #43222, #47469, #4916 ) ;
#20963=DIRECTION ( 'NONE',  ( -0.000000000000000000, 0.000000000000000000, 1.000000000000000000 ) ) ;
#20973=ORIENTED_EDGE ( 'NONE', *, *, #5607, .T. ) ;
#20996=ORIENTED_EDGE ( 'NONE', *, *, #1850, .T. ) ;
#21092=DIRECTION ( 'NONE',  ( 0.000000000000000000, -0.9999993111447558203, 0.001173758924898823551 ) ) ;
#21121=CARTESIAN_POINT ( 'NONE',  ( 410.0000000000000000, 190.0000000000000000, 0.000000000000000000 ) ) ;
#21129=CARTESIAN_POINT ( 'NONE',  ( -22.50000000000000355, 207.5000000000000284, 20.00000000000000000 ) ) ;
#21132=SURFACE_SIDE_STYLE ('',( #69306 ) ) ;
#21134=ORIENTED_EDGE ( 'NONE', *, *, #66760, .T. ) ;
#21135=EDGE_CURVE ( 'NONE', #59365, #28423, #5916, .T. ) ;
#21187=DIRECTION ( 'NONE',  ( -0.000000000000000000, -0.000000000000000000, -1.000000000000000000 ) ) ;
#21190=EDGE_CURVE ( 'NONE', #41559, #54229, #47498, .T. ) ;
#21244=ORIENTED_EDGE ( 'NONE', *, *, #16902, .T. ) ;
#21260=DIRECTION ( 'NONE',  ( -0.000000000000000000, -1.000000000000000000, -0.000000000000000000 ) ) ;
#21338=FACE_OUTER_BOUND ( 'NONE', #63270, .T. ) ;
#21340=CARTESIAN_POINT ( 'NONE',  ( 99.71998884745383407, 190.0000000000000000, 7.478223336038896996 ) ) ;
#21343=EDGE_CURVE ( 'NONE', #61832, #28258, #27299, .T. ) ;
#21404=ADVANCED_BREP_SHAPE_REPRESENTATION ( '', ( #65110, #18036, #66832 ), #17430 ) ;
#21502=LINE ( 'NONE', #16229, #45626 ) ;
#21507=LINE ( 'NONE', #26797, #52044 ) ;
#21515=CARTESIAN_POINT ( 'NONE',  ( 410.0000000000000000, 0.000000000000000000, 0.000000000000000000 ) ) ;
#21517=VECTOR ( 'NONE', #29572, 1000.000000000000227 ) ;
#21556=LINE ( 'NONE', #42672, #47852 ) ;
#21615=LINE ( 'NONE', #27938, #56259 ) ;
#21738=ORIENTED_EDGE ( 'NONE', *, *, #46200, .T. ) ;
#21902=EDGE_LOOP ( 'NONE', ( #26574, #45100, #58690, #42968, #31610, #13468, #38650, #35437 ) ) ;
#21949=CARTESIAN_POINT ( 'NONE',  ( 47.74291447196797833, 2.000000000000001776, -75.60236247897087480 ) ) ;
#22114=CYLINDRICAL_SURFACE ( 'NONE', #51668, 91.99999999999997158 ) ;
#22168=CARTESIAN_POINT ( 'NONE',  ( -35.00000000000000000, -35.00000000000000000, 0.000000000000000000 ) ) ;
#22193=AXIS2_PLACEMENT_3D ( 'NONE', #13526, #18452, #13183 ) ;
#22219=FACE_OUTER_BOUND ( 'NONE', #1068, .T. ) ;
#22270=CARTESIAN_POINT ( 'NONE',  ( -35.00000000000000000, 225.0000000000000000, 0.000000000000000000 ) ) ;
#22291=EDGE_LOOP ( 'NONE', ( #17970, #27405, #69147, #22307 ) ) ;
#22307=ORIENTED_EDGE ( 'NONE', *, *, #65368, .T. ) ;
#22328=DIRECTION ( 'NONE',  ( 0.000000000000000000, 0.000000000000000000, -1.000000000000000000 ) ) ;
#22330=EDGE_CURVE ( 'NONE', #26863, #8775, #17226, .T. ) ;
#22373=ORIENTED_EDGE ( 'NONE', *, *, #29287, .T. ) ;
#22374=VERTEX_POINT ( 'NONE', #66716 ) ;
#22463=CARTESIAN_POINT ( 'NONE',  ( 410.0000000000000000, 190.0000000000000000, -90.00000000000000000 ) ) ;
#22474=LINE ( 'NONE', #43913, #9657 ) ;
#22615=ADVANCED_FACE ( 'NONE', ( #11747 ), #1921, .F. ) ;
#22680=DIRECTION ( 'NONE',  ( 0.000000000000000000, 0.000000000000000000, -1.000000000000000000 ) ) ;
#22712=VERTEX_POINT ( 'NONE', #36692 ) ;
#22742=LINE ( 'NONE', #28009, #25147 ) ;
#22839=CARTESIAN_POINT ( 'NONE',  ( 122.2516123306975402, 190.0000000000000000, -91.28179539054376335 ) ) ;
#22881=ORIENTED_EDGE ( 'NONE', *, *, #67167, .F. ) ;
#22913=FACE_BOUND ( 'NONE', #55951, .T. ) ;
#22935=DIRECTION ( 'NONE',  ( 0.3962817440048566620, 0.9137562205704280460, -0.08950055160341972849 ) ) ;
#23089=EDGE_CURVE ( 'NONE', #61986, #32859, #61938, .T. ) ;
#23136=EDGE_CURVE ( 'NONE', #43935, #61832, #66774, .T. ) ;
#23162=VECTOR ( 'NONE', #65313, 1000.000000000000000 ) ;
#23198=VERTEX_POINT ( 'NONE', #21121 ) ;
#23266=DIRECTION ( 'NONE',  ( 0.000000000000000000, 0.000000000000000000, -1.000000000000000000 ) ) ;
#23274=VECTOR ( 'NONE', #66468, 1000.000000000000000 ) ;
#23286=CARTESIAN_POINT ( 'NONE',  ( 0.000000000000000000, 500.0000000000000000, 0.000000000000000000 ) ) ;
#23334=CARTESIAN_POINT ( 'NONE',  ( 324.1677456657756125, 188.0000000000000000, -123.1183350412580779 ) ) ;
#23374=CARTESIAN_POINT ( 'NONE',  ( 0.000000000000000000, -0.1068809833119260672, -91.05865558859387932 ) ) ;
#23378=AXIS2_PLACEMENT_3D ( 'NONE', #65414, #17206, #38679 ) ;
#23384=VECTOR ( 'NONE', #15865, 1000.000000000000000 ) ;
#23418=CIRCLE ( 'NONE', #68351, 5.000000000000000888 ) ;
#23428=EDGE_LOOP ( 'NONE', ( #68713, #25660 ) ) ;
#23457=EDGE_CURVE ( 'NONE', #6944, #38976, #40944, .T. ) ;
#23467=DIRECTION ( 'NONE',  ( -0.000000000000000000, -0.000000000000000000, -1.000000000000000000 ) ) ;
#23556=VERTEX_POINT ( 'NONE', #48210 ) ;
#23595=ORIENTED_EDGE ( 'NONE', *, *, #22330, .F. ) ;
#23618=DIRECTION ( 'NONE',  ( 0.000000000000000000, -0.000000000000000000, 1.000000000000000000 ) ) ;
#23623=CARTESIAN_POINT ( 'NONE',  ( -22.50000000000000355, -17.50000000000000000, 1.999999999999998224 ) ) ;
#23755=CYLINDRICAL_SURFACE ( 'NONE', #31438, 5.000000000000004441 ) ;
#23798=VECTOR ( 'NONE', #52743, 1000.000000000000000 ) ;
#23831=ADVANCED_FACE ( 'NONE', ( #28024 ), #32276, .T. ) ;
#23867=DIRECTION ( 'NONE',  ( -0.000000000000000000, -1.000000000000000000, -0.000000000000000000 ) ) ;
#23874=CARTESIAN_POINT ( 'NONE',  ( 410.0000000000000000, 0.000000000000000000, 2.000000000000000000 ) ) ;
#23875=DIRECTION ( 'NONE',  ( -1.000000000000000000, 0.000000000000000000, 0.000000000000000000 ) ) ;
#23917=CARTESIAN_POINT ( 'NONE',  ( -12.50000000000000000, 207.5000000000000284, 20.00000000000000000 ) ) ;
#23963=ORIENTED_EDGE ( 'NONE', *, *, #27948, .T. ) ;
#23999=ORIENTED_EDGE ( 'NONE', *, *, #61245, .T. ) ;
#24096=DIRECTION ( 'NONE',  ( -1.000000000000000000, 0.000000000000000000, 0.000000000000000000 ) ) ;
#24134=AXIS2_PLACEMENT_3D ( 'NONE', #18603, #28816, #66810 ) ;
#24141=DIRECTION ( 'NONE',  ( -0.000000000000000000, -0.000000000000000000, -1.000000000000000000 ) ) ;
#24153=ORIENTED_EDGE ( 'NONE', *, *, #68245, .T. ) ;
#24193=VERTEX_POINT ( 'NONE', #28649 ) ;
#24254=EDGE_LOOP ( 'NONE', ( #19158, #58420, #25715, #22881, #17747, #12193 ) ) ;
#24321=DIRECTION ( 'NONE',  ( -1.000000000000000000, 0.000000000000000000, 0.000000000000000000 ) ) ;
#24356=LINE ( 'NONE', #34908, #13773 ) ;
#24448=PLANE ( 'NONE',  #63772 ) ;
#24524=ORIENTED_EDGE ( 'NONE', *, *, #62082, .F. ) ;
#24525=FACE_BOUND ( 'NONE', #68964, .T. ) ;
#24575=AXIS2_PLACEMENT_3D ( 'NONE', #6759, #1139, #28208 ) ;
#24618=EDGE_CURVE ( 'NONE', #15622, #44112, #60107, .T. ) ;
#24640=EDGE_CURVE ( 'NONE', #50057, #34560, #33683, .T. ) ;
#24663=CIRCLE ( 'NONE', #63958, 299.9999999999999432 ) ;
#24717=LINE ( 'NONE', #57403, #16805 ) ;
#24746=CARTESIAN_POINT ( 'NONE',  ( 563.4809901518626702, 190.0000000000000000, 57.79371821540657095 ) ) ;
#24785=CARTESIAN_POINT ( 'NONE',  ( 99.71998884745383407, 2.000000000000000000, 7.478223336038896996 ) ) ;
#24847=VECTOR ( 'NONE', #49152, 1000.000000000000000 ) ;
#24859=FACE_OUTER_BOUND ( 'NONE', #4274, .T. ) ;
#24876=ORIENTED_EDGE ( 'NONE', *, *, #31851, .F. ) ;
#24899=ORIENTED_EDGE ( 'NONE', *, *, #45762, .F. ) ;
#24905=FACE_OUTER_BOUND ( 'NONE', #4800, .T. ) ;
#24954=CIRCLE ( 'NONE', #66393, 300.0000000000000000 ) ;
#25024=VERTEX_POINT ( 'NONE', #50461 ) ;
#25029=EDGE_CURVE ( 'NONE', #31022, #55566, #49739, .T. ) ;
#25048=VERTEX_POINT ( 'NONE', #2618 ) ;
#25085=ORIENTED_EDGE ( 'NONE', *, *, #2634, .T. ) ;
#25086=FACE_OUTER_BOUND ( 'NONE', #32574, .T. ) ;
#25103=VECTOR ( 'NONE', #47487, 1000.000000000000000 ) ;
#25147=VECTOR ( 'NONE', #24141, 1000.000000000000000 ) ;
#25269=CARTESIAN_POINT ( 'NONE',  ( 262.2516123306975260, 190.0000000000000000, -91.28179539054376335 ) ) ;
#25331=DIRECTION ( 'NONE',  ( -0.000000000000000000, -0.000000000000000000, -1.000000000000000000 ) ) ;
#25341=AXIS2_PLACEMENT_3D ( 'NONE', #23286, #44731, #17999 ) ;
#25416=CARTESIAN_POINT ( 'NONE',  ( 311.8713128290285113, 188.0000000000000000, -151.4173447659616443 ) ) ;
#25515=LINE ( 'NONE', #35020, #46374 ) ;
#25538=VECTOR ( 'NONE', #18984, 1000.000000000000000 ) ;
#25583=CIRCLE ( 'NONE', #34580, 5.000000000000004441 ) ;
#25660=ORIENTED_EDGE ( 'NONE', *, *, #29287, .F. ) ;
#25694=CARTESIAN_POINT ( 'NONE',  ( 422.4999999999999432, 207.5000000000000284, 0.000000000000000000 ) ) ;
#25715=ORIENTED_EDGE ( 'NONE', *, *, #37030, .F. ) ;
#25759=ORIENTED_EDGE ( 'NONE', *, *, #13168, .F. ) ;
#25844=ORIENTED_EDGE ( 'NONE', *, *, #29862, .F. ) ;
#25888=EDGE_LOOP ( 'NONE', ( #58484, #63953, #22373, #1120 ) ) ;
#25946=ORIENTED_EDGE ( 'NONE', *, *, #1016, .F. ) ;
#26033=LINE ( 'NONE', #57699, #23798 ) ;
#26038=EDGE_LOOP ( 'NONE', ( #47584, #50216, #24524, #3079 ) ) ;
#26043=ORIENTED_EDGE ( 'NONE', *, *, #51492, .T. ) ;
#26048=PLANE ( 'NONE',  #855 ) ;
#26191=EDGE_LOOP ( 'NONE', ( #31822, #43272, #20732, #25085 ) ) ;
#26192=ORIENTED_EDGE ( 'NONE', *, *, #28005, .F. ) ;
#26236=EDGE_CURVE ( 'NONE', #22374, #16361, #21556, .T. ) ;
#26290=ORIENTED_EDGE ( 'NONE', *, *, #25029, .T. ) ;
#26396=DIRECTION ( 'NONE',  ( 0.000000000000000000, 0.000000000000000000, -1.000000000000000000 ) ) ;
#26414=CARTESIAN_POINT ( 'NONE',  ( 0.000000000000000000, 190.0000000000000000, 0.000000000000000000 ) ) ;
#26440=CARTESIAN_POINT ( 'NONE',  ( 99.71998884745383407, 188.0000000000000000, 0.000000000000000000 ) ) ;
#26511=VERTEX_POINT ( 'NONE', #57392 ) ;
#26566=CIRCLE ( 'NONE', #34474, 299.9999999999999432 ) ;
#26574=ORIENTED_EDGE ( 'NONE', *, *, #46200, .F. ) ;
#26580=ORIENTED_EDGE ( 'NONE', *, *, #627, .T. ) ;
#26594=EDGE_CURVE ( 'NONE', #62220, #26511, #67610, .T. ) ;
#26622=EDGE_CURVE ( 'NONE', #54229, #29750, #15876, .T. ) ;
#26684=EDGE_CURVE ( 'NONE', #28328, #6711, #31711, .T. ) ;
#26778=DIRECTION ( 'NONE',  ( -0.3738650651659383151, 0.9230658208099267181, -0.09041240789275073464 ) ) ;
#26797=CARTESIAN_POINT ( 'NONE',  ( -3.306248862503413655, 500.0000000000000000, -91.64566090791306863 ) ) ;
#26863=VERTEX_POINT ( 'NONE', #56994 ) ;
#27035=DIRECTION ( 'NONE',  ( -0.000000000000000000, -1.000000000000000000, 0.000000000000000000 ) ) ;
#27047=VECTOR ( 'NONE', #16153, 1000.000000000000000 ) ;
#27124=VECTOR ( 'NONE', #47441, 1000.000000000000000 ) ;
#27215=DIRECTION ( 'NONE',  ( -0.000000000000000000, -0.000000000000000000, -1.000000000000000000 ) ) ;
#27232=EDGE_CURVE ( 'NONE', #61740, #66549, #31140, .T. ) ;
#27260=EDGE_LOOP ( 'NONE', ( #17708, #51712, #2931, #28767 ) ) ;
#27270=VERTEX_POINT ( 'NONE', #48652 ) ;
#27299=LINE ( 'NONE', #27650, #37411 ) ;
#27401=ORIENTED_EDGE ( 'NONE', *, *, #26594, .T. ) ;
#27405=ORIENTED_EDGE ( 'NONE', *, *, #51492, .F. ) ;
#27498=CARTESIAN_POINT ( 'NONE',  ( 450.2085304802404835, 2.000000000000001776, -219.9999999999999147 ) ) ;
#27537=ADVANCED_FACE ( 'NONE', ( #25086 ), #46523, .F. ) ;
#27602=ORIENTED_EDGE ( 'NONE', *, *, #63589, .F. ) ;
#27607=VERTEX_POINT ( 'NONE', #14858 ) ;
#27650=CARTESIAN_POINT ( 'NONE',  ( 0.000000000000000000, 190.0000000000000000, 0.000000000000000000 ) ) ;
#27876=EDGE_LOOP ( 'NONE', ( #37829, #10159 ) ) ;
#27885=EDGE_CURVE ( 'NONE', #50879, #45198, #42186, .T. ) ;
#27911=DIRECTION ( 'NONE',  ( -0.3754025596372949636, 0.9268618657695261165, 0.000000000000000000 ) ) ;
#27928=EDGE_LOOP ( 'NONE', ( #68295, #57501, #39849, #49530 ) ) ;
#27938=CARTESIAN_POINT ( 'NONE',  ( 410.0000000000000000, 190.0000000000000000, 0.000000000000000000 ) ) ;
#27948=EDGE_CURVE ( 'NONE', #58197, #59365, #66967, .T. ) ;
#28005=EDGE_CURVE ( 'NONE', #65415, #2294, #655, .T. ) ;
#28009=CARTESIAN_POINT ( 'NONE',  ( -22.50000000000000355, -17.50000000000000000, 20.00000000000000000 ) ) ;
#28024=FACE_OUTER_BOUND ( 'NONE', #64026, .T. ) ;
#28029=EDGE_CURVE ( 'NONE', #1594, #60452, #22474, .T. ) ;
#28031=EDGE_LOOP ( 'NONE', ( #50504, #21134, #35510, #3528 ) ) ;
#28035=DIRECTION ( 'NONE',  ( -0.000000000000000000, -1.000000000000000000, 0.000000000000000000 ) ) ;
#28089=ADVANCED_FACE ( 'NONE', ( #14009 ), #50257, .F. ) ;
#28181=CARTESIAN_POINT ( 'NONE',  ( 311.8713128290285113, 190.0000000000000000, 346.5826552340383842 ) ) ;
#28206=PLANE ( 'NONE',  #34430 ) ;
#28208=DIRECTION ( 'NONE',  ( 0.000000000000000000, 0.000000000000000000, -1.000000000000000000 ) ) ;
#28209=CARTESIAN_POINT ( 'NONE',  ( 0.000000000000000000, -0.1068809833119260672, -91.05865558859387932 ) ) ;
#28231=EDGE_CURVE ( 'NONE', #61740, #18178, #12624, .T. ) ;
#28258=VERTEX_POINT ( 'NONE', #20317 ) ;
#28281=CARTESIAN_POINT ( 'NONE',  ( -35.00000000000000000, 225.0000000000000000, 2.000000000000000000 ) ) ;
#28328=VERTEX_POINT ( 'NONE', #25269 ) ;
#28374=LINE ( 'NONE', #1301, #56498 ) ;
#28406=ORIENTED_EDGE ( 'NONE', *, *, #10921, .F. ) ;
#28423=VERTEX_POINT ( 'NONE', #55090 ) ;
#28424=EDGE_CURVE ( 'NONE', #55566, #56923, #33661, .T. ) ;
#28448=DIRECTION ( 'NONE',  ( 0.000000000000000000, 0.000000000000000000, -1.000000000000000000 ) ) ;
#28478=VERTEX_POINT ( 'NONE', #17100 ) ;
#28649=CARTESIAN_POINT ( 'NONE',  ( 396.6937511374966334, 500.0000000000000000, -51.64566090791306863 ) ) ;
#28712=DIRECTION ( 'NONE',  ( -0.000000000000000000, -1.000000000000000000, -0.000000000000000000 ) ) ;
#28767=ORIENTED_EDGE ( 'NONE', *, *, #1016, .T. ) ;
#28773=LINE ( 'NONE', #11522, #24847 ) ;
#28816=DIRECTION ( 'NONE',  ( 0.000000000000000000, 0.000000000000000000, -1.000000000000000000 ) ) ;
#28823=CARTESIAN_POINT ( 'NONE',  ( 450.2085304802404266, 190.0000000000000000, -250.0000000000000000 ) ) ;
#28963=ORIENTED_EDGE ( 'NONE', *, *, #12905, .T. ) ;
#28972=DIRECTION ( 'NONE',  ( -0.000000000000000000, -1.000000000000000000, -0.000000000000000000 ) ) ;
#29000=UNCERTAINTY_MEASURE_WITH_UNIT (LENGTH_MEASURE( 1.000000000000000082E-05 ), #46628, 'distance_accuracy_value', 'NONE');
#29023=FACE_OUTER_BOUND ( 'NONE', #64242, .T. ) ;
#29031=DIRECTION ( 'NONE',  ( -1.048079516971690241E-11, 0.000000000000000000, -1.000000000000000000 ) ) ;
#29048=ORIENTED_EDGE ( 'NONE', *, *, #45762, .T. ) ;
#29059=FACE_OUTER_BOUND ( 'NONE', #52208, .T. ) ;
#29141=CARTESIAN_POINT ( 'NONE',  ( 259.2042601260359334, 188.0000000000000000, -23.09547038499562888 ) ) ;
#29150=CARTESIAN_POINT ( 'NONE',  ( 410.0000000000000000, 190.0000000000000000, 2.000000000000000000 ) ) ;
#29215=CARTESIAN_POINT ( 'NONE',  ( 427.4999999999999432, -17.50000000000000000, 1.999999999999998224 ) ) ;
#29277=DIRECTION ( 'NONE',  ( -0.000000000000000000, -0.000000000000000000, -1.000000000000000000 ) ) ;
#29287=EDGE_CURVE ( 'NONE', #29750, #8207, #58058, .T. ) ;
#29375=EDGE_CURVE ( 'NONE', #28328, #52426, #604, .T. ) ;
#29555=AXIS2_PLACEMENT_3D ( 'NONE', #12972, #23867, #45310 ) ;
#29572=DIRECTION ( 'NONE',  ( 0.3962817440048567175, 0.9137562205704280460, -0.08950055160341974236 ) ) ;
#29638=EDGE_CURVE ( 'NONE', #38509, #23556, #14021, .T. ) ;
#29657=ORIENTED_EDGE ( 'NONE', *, *, #3064, .F. ) ;
#29696=PLANE ( 'NONE',  #45715 ) ;
#29708=ADVANCED_FACE ( 'NONE', ( #2432 ), #50614, .T. ) ;
#29712=EDGE_CURVE ( 'NONE', #61832, #17233, #19642, .T. ) ;
#29750=VERTEX_POINT ( 'NONE', #13674 ) ;
#29754=LINE ( 'NONE', #69368, #64486 ) ;
#29784=FACE_BOUND ( 'NONE', #3069, .T. ) ;
#29824=DIRECTION ( 'NONE',  ( 1.000000000000000000, 0.000000000000000000, 0.000000000000000000 ) ) ;
#29826=DIRECTION ( 'NONE',  ( 0.000000000000000000, 1.000000000000000000, -0.000000000000000000 ) ) ;
#29862=EDGE_CURVE ( 'NONE', #28258, #30681, #4185, .T. ) ;
#29996=ADVANCED_FACE ( 'NONE', ( #9440 ), #57630, .F. ) ;
#30053=FACE_OUTER_BOUND ( 'NONE', #65926, .T. ) ;
#30179=CARTESIAN_POINT ( 'NONE',  ( 99.71998884745383407, 188.0000000000000000, 7.478223336038896996 ) ) ;
#30337=EDGE_CURVE ( 'NONE', #8207, #29750, #25583, .T. ) ;
#30422=ORIENTED_EDGE ( 'NONE', *, *, #40565, .T. ) ;
#30425=DIRECTION ( 'NONE',  ( -0.000000000000000000, 0.000000000000000000, 1.000000000000000000 ) ) ;
#30477=DIRECTION ( 'NONE',  ( -0.000000000000000000, 0.000000000000000000, 1.000000000000000000 ) ) ;
#30552=AXIS2_PLACEMENT_3D ( 'NONE', #28209, #17671, #66228 ) ;
#30638=VERTEX_POINT ( 'NONE', #65064 ) ;
#30639=CARTESIAN_POINT ( 'NONE',  ( 427.4999999999999432, 207.5000000000000284, 0.000000000000000000 ) ) ;
#30681=VERTEX_POINT ( 'NONE', #39726 ) ;
#30722=ADVANCED_FACE ( 'NONE', ( #43934 ), #5957, .T. ) ;
#30753=CARTESIAN_POINT ( 'NONE',  ( 427.4999999999999432, -17.50000000000000000, 20.00000000000000000 ) ) ;
#30864=DIRECTION ( 'NONE',  ( 1.000000000000000000, 0.000000000000000000, 0.000000000000000000 ) ) ;
#30896=DIRECTION ( 'NONE',  ( 0.000000000000000000, -1.000000000000000000, 0.000000000000000000 ) ) ;
#31022=VERTEX_POINT ( 'NONE', #57209 ) ;
#31140=LINE ( 'NONE', #10020, #9612 ) ;
#31151=ORIENTED_EDGE ( 'NONE', *, *, #22330, .T. ) ;
#31153=AXIS2_PLACEMENT_3D ( 'NONE', #45765, #24321, #39791 ) ;
#31220=LINE ( 'NONE', #52651, #32308 ) ;
#31290=EDGE_CURVE ( 'NONE', #30681, #38509, #52525, .T. ) ;
#31312=ORIENTED_EDGE ( 'NONE', *, *, #68526, .F. ) ;
#31323=ORIENTED_EDGE ( 'NONE', *, *, #23136, .T. ) ;
#31438=AXIS2_PLACEMENT_3D ( 'NONE', #61723, #60687, #55765 ) ;
#31489=AXIS2_PLACEMENT_3D ( 'NONE', #45105, #34221, #18039 ) ;
#31491=CARTESIAN_POINT ( 'NONE',  ( 0.000000000000000000, 0.000000000000000000, 2.000000000000000000 ) ) ;
#31610=ORIENTED_EDGE ( 'NONE', *, *, #29638, .F. ) ;
#31696=EDGE_CURVE ( 'NONE', #43800, #28328, #13016, .T. ) ;
#31708=LINE ( 'NONE', #26440, #50086 ) ;
#31711=LINE ( 'NONE', #10249, #32041 ) ;
#31764=VECTOR ( 'NONE', #65285, 1000.000000000000000 ) ;
#31779=CYLINDRICAL_SURFACE ( 'NONE', #59189, 5.000000000000004441 ) ;
#31822=ORIENTED_EDGE ( 'NONE', *, *, #35435, .F. ) ;
#31851=EDGE_CURVE ( 'NONE', #15622, #38606, #18973, .T. ) ;
#31933=DIRECTION ( 'NONE',  ( 0.000000000000000000, 0.000000000000000000, -1.000000000000000000 ) ) ;
#31944=DIRECTION ( 'NONE',  ( -0.000000000000000000, 0.000000000000000000, 1.000000000000000000 ) ) ;
#32041=VECTOR ( 'NONE', #63031, 1000.000000000000000 ) ;
#32080=DIRECTION ( 'NONE',  ( 0.000000000000000000, 0.000000000000000000, -1.000000000000000000 ) ) ;
#32085=CARTESIAN_POINT ( 'NONE',  ( 450.2085304802404266, 188.0000000000000000, 7.478223336038896996 ) ) ;
#32196=EDGE_LOOP ( 'NONE', ( #41412, #14368, #18494, #19792, #48066, #21738, #62188, #62840, #49779 ) ) ;
#32220=DIRECTION ( 'NONE',  ( -1.048079516971690241E-11, 0.000000000000000000, -1.000000000000000000 ) ) ;
#32240=CARTESIAN_POINT ( 'NONE',  ( 0.000000000000000000, 0.000000000000000000, 0.000000000000000000 ) ) ;
#32274=ORIENTED_EDGE ( 'NONE', *, *, #41999, .F. ) ;
#32276=PLANE ( 'NONE',  #7305 ) ;
#32308=VECTOR ( 'NONE', #68163, 1000.000000000000000 ) ;
#32341=ORIENTED_EDGE ( 'NONE', *, *, #11548, .F. ) ;
#32353=DIRECTION ( 'NONE',  ( -0.000000000000000000, -0.000000000000000000, -1.000000000000000000 ) ) ;
#32389=ORIENTED_EDGE ( 'NONE', *, *, #12905, .F. ) ;
#32449=CARTESIAN_POINT ( 'NONE',  ( 422.4999999999999432, 207.5000000000000284, 1.999999999999998224 ) ) ;
#32467=DIRECTION ( 'NONE',  ( -0.3754023374827052950, 0.9268613172740186590, -0.001087912492708085609 ) ) ;
#32540=EDGE_LOOP ( 'NONE', ( #32832, #7291, #46023, #3080 ) ) ;
#32544=EDGE_CURVE ( 'NONE', #2294, #65415, #18944, .T. ) ;
#32559=CARTESIAN_POINT ( 'NONE',  ( 311.8713128290285113, 188.0000000000000000, 346.5826552340383842 ) ) ;
#32574=EDGE_LOOP ( 'NONE', ( #48315, #46174, #11789, #26580 ) ) ;
#32632=EDGE_CURVE ( 'NONE', #19572, #53112, #54924, .T. ) ;
#32690=CARTESIAN_POINT ( 'NONE',  ( 311.9732115134679020, 188.0000000000000000, -151.4173343409194672 ) ) ;
#32823=DIRECTION ( 'NONE',  ( -1.000000000000000000, 0.000000000000000000, 0.000000000000000000 ) ) ;
#32832=ORIENTED_EDGE ( 'NONE', *, *, #18750, .F. ) ;
#32852=AXIS2_PLACEMENT_3D ( 'NONE', #44701, #33799, #7063 ) ;
#32859=VERTEX_POINT ( 'NONE', #2549 ) ;
#32938=EDGE_CURVE ( 'NONE', #27607, #50057, #19066, .T. ) ;
#32958=VECTOR ( 'NONE', #48450, 1000.000000000000000 ) ;
#33001=EDGE_LOOP ( 'NONE', ( #46038, #62130, #29048, #44251 ) ) ;
#33006=EDGE_CURVE ( 'NONE', #16361, #30638, #6657, .T. ) ;
#33227=DIRECTION ( 'NONE',  ( 0.000000000000000000, -0.9999993111447558203, 0.001173758924898823551 ) ) ;
#33238=DIRECTION ( 'NONE',  ( -0.000000000000000000, 0.000000000000000000, 1.000000000000000000 ) ) ;
#33310=CARTESIAN_POINT ( 'NONE',  ( 444.9999999999999432, -35.00000000000000000, 2.000000000000000000 ) ) ;
#33323=VERTEX_POINT ( 'NONE', #56490 ) ;
#33353=ADVANCED_FACE ( 'NONE', ( #40278 ), #23755, .F. ) ;
#33365=LINE ( 'NONE', #49863, #46408 ) ;
#33386=CARTESIAN_POINT ( 'NONE',  ( 260.0716287634991204, 189.9999999999999432, -91.28179539054374914 ) ) ;
#33393=DIRECTION ( 'NONE',  ( 0.000000000000000000, 0.000000000000000000, -1.000000000000000000 ) ) ;
#33478=CARTESIAN_POINT ( 'NONE',  ( 410.0000000000000000, 2.000000000000001776, -90.00000000000000000 ) ) ;
#33593=EDGE_LOOP ( 'NONE', ( #39521, #63928, #65761, #60754, #34653, #40843, #17737, #5753, #17597 ) ) ;
#33640=CARTESIAN_POINT ( 'NONE',  ( 2.005731055991735623, 188.0000000000000000, 0.000000000000000000 ) ) ;
#33647=VECTOR ( 'NONE', #30864, 1000.000000000000000 ) ;
#33661=LINE ( 'NONE', #38222, #23162 ) ;
#33683=LINE ( 'NONE', #37549, #36530 ) ;
#33751=ORIENTED_EDGE ( 'NONE', *, *, #26684, .F. ) ;
#33799=DIRECTION ( 'NONE',  ( -1.000000000000000000, 0.000000000000000000, 0.000000000000000000 ) ) ;
#33804=EDGE_CURVE ( 'NONE', #8775, #2294, #24717, .T. ) ;
#33957=CARTESIAN_POINT ( 'NONE',  ( 324.1677456657756125, 2.000000000000000000, -123.1183350412580779 ) ) ;
#34078=ORIENTED_EDGE ( 'NONE', *, *, #31696, .T. ) ;
#34107=ORIENTED_EDGE ( 'NONE', *, *, #58658, .T. ) ;
#34145=ADVANCED_FACE ( 'NONE', ( #34845 ), #19000, .F. ) ;
#34221=DIRECTION ( 'NONE',  ( 0.000000000000000000, -1.000000000000000000, 0.000000000000000000 ) ) ;
#34285=CIRCLE ( 'NONE', #54481, 498.0000000000000000 ) ;
#34290=CYLINDRICAL_SURFACE ( 'NONE', #18402, 89.99999999999997158 ) ;
#34315=LINE ( 'NONE', #39924, #7611 ) ;
#34326=VECTOR ( 'NONE', #40253, 1000.000000000000000 ) ;
#34405=EDGE_CURVE ( 'NONE', #33323, #39735, #41503, .T. ) ;
#34430=AXIS2_PLACEMENT_3D ( 'NONE', #51331, #62213, #54226 ) ;
#34474=AXIS2_PLACEMENT_3D ( 'NONE', #64683, #27035, #52732 ) ;
#34530=VECTOR ( 'NONE', #61850, 1000.000000000000000 ) ;
#34560=VERTEX_POINT ( 'NONE', #32240 ) ;
#34580=AXIS2_PLACEMENT_3D ( 'NONE', #30639, #35572, #13763 ) ;
#34608=ORIENTED_EDGE ( 'NONE', *, *, #32544, .T. ) ;
#34643=AXIS2_PLACEMENT_3D ( 'NONE', #5759, #64165, #65212 ) ;
#34653=ORIENTED_EDGE ( 'NONE', *, *, #68543, .F. ) ;
#34720=AXIS2_PLACEMENT_3D ( 'NONE', #62411, #35689, #24096 ) ;
#34798=DIRECTION ( 'NONE',  ( 0.000000000000000000, 1.000000000000000000, -0.000000000000000000 ) ) ;
#34809=CARTESIAN_POINT ( 'NONE',  ( 173.0237957311180708, 69.97204739562489806, -91.14091141288837150 ) ) ;
#34845=FACE_OUTER_BOUND ( 'NONE', #16971, .T. ) ;
#34870=FACE_OUTER_BOUND ( 'NONE', #21902, .T. ) ;
#34885=AXIS2_PLACEMENT_3D ( 'NONE', #4399, #21260, #58881 ) ;
#34908=CARTESIAN_POINT ( 'NONE',  ( 396.6937511374966334, 500.0000000000000000, -51.64566090791306863 ) ) ;
#34913=ORIENTED_EDGE ( 'NONE', *, *, #41139, .F. ) ;
#34946=DIRECTION ( 'NONE',  ( -1.000000000000000000, 0.000000000000000000, 0.000000000000000000 ) ) ;
#34954=EDGE_LOOP ( 'NONE', ( #4773, #43606, #61868, #34078 ) ) ;
#34955=ORIENTED_EDGE ( 'NONE', *, *, #24640, .T. ) ;
#34957=LINE ( 'NONE', #2597, #18447 ) ;
#35020=CARTESIAN_POINT ( 'NONE',  ( -1.148430018225575555, 500.0000000000000000, -0.000000000000000000 ) ) ;
#35028=VECTOR ( 'NONE', #57227, 1000.000000000000000 ) ;
#35115=DIRECTION ( 'NONE',  ( -0.000000000000000000, -1.000000000000000000, -0.000000000000000000 ) ) ;
#35138=AXIS2_PLACEMENT_3D ( 'NONE', #1267, #18147, #16740 ) ;
#35239=LINE ( 'NONE', #13103, #42678 ) ;
#35272=CARTESIAN_POINT ( 'NONE',  ( 122.2516123306975402, 190.0000000000000000, -21.28179539054375624 ) ) ;
#35277=AXIS2_PLACEMENT_3D ( 'NONE', #12055, #49320, #38797 ) ;
#35339=CARTESIAN_POINT ( 'NONE',  ( 122.2516123306975402, 190.0000000000000000, -91.28179539054376335 ) ) ;
#35435=EDGE_CURVE ( 'NONE', #38900, #19572, #42736, .T. ) ;
#35437=ORIENTED_EDGE ( 'NONE', *, *, #9138, .T. ) ;
#35481=DIRECTION ( 'NONE',  ( -0.000000000000000000, -1.000000000000000000, -0.000000000000000000 ) ) ;
#35510=ORIENTED_EDGE ( 'NONE', *, *, #51660, .F. ) ;
#35572=DIRECTION ( 'NONE',  ( 0.000000000000000000, 0.000000000000000000, -1.000000000000000000 ) ) ;
#35626=AXIS2_PLACEMENT_3D ( 'NONE', #41519, #52071, #3887 ) ;
#35682=FILL_AREA_STYLE_COLOUR ( '', #51633 ) ;
#35689=DIRECTION ( 'NONE',  ( 0.000000000000000000, 0.000000000000000000, -1.000000000000000000 ) ) ;
#35773=VECTOR ( 'NONE', #61867, 1000.000000000000000 ) ;
#35780=ADVANCED_FACE ( 'NONE', ( #58533 ), #46962, .F. ) ;
#35804=DIRECTION ( 'NONE',  ( 1.000000000000000000, 0.000000000000000000, -0.000000000000000000 ) ) ;
#35828=CARTESIAN_POINT ( 'NONE',  ( 311.8713128290285113, 2.000000000000001776, -151.4173447659616443 ) ) ;
#35865=CARTESIAN_POINT ( 'NONE',  ( 544.6745185807129701, 0.000000000000000000, 34.73878747406611467 ) ) ;
#35896=APPLICATION_CONTEXT ( 'automotive_design' ) ;
#35948=EDGE_CURVE ( 'NONE', #11952, #24193, #54994, .T. ) ;
#36163=ADVANCED_FACE ( 'NONE', ( #56395 ), #62371, .F. ) ;
#36171=DIRECTION ( 'NONE',  ( -0.000000000000000000, -1.000000000000000000, 0.000000000000000000 ) ) ;
#36198=CLOSED_SHELL ( 'NONE', ( #18520, #69221, #1590, #46587, #59694, #22615, #61380, #54613, #36163, #14069, #30722, #1663, #61453, #38163, #6757, #37707, #7881, #29708, #13665, #11926, #13820, #35780, #52871, #11799, #50385, #60735, #19859, #23831 ) ) ;
#36208=ORIENTED_EDGE ( 'NONE', *, *, #40565, .F. ) ;
#36233=DIRECTION ( 'NONE',  ( -0.000000000000000000, 0.001173758924898823768, 0.9999993111447559313 ) ) ;
#36243=CYLINDRICAL_SURFACE ( 'NONE', #1944, 97.99999999999994316 ) ;
#36359=EDGE_LOOP ( 'NONE', ( #26192, #12777 ) ) ;
#36457=LINE ( 'NONE', #45633, #35028 ) ;
#36518=EDGE_CURVE ( 'NONE', #28258, #11580, #21615, .T. ) ;
#36530=VECTOR ( 'NONE', #967, 1000.000000000000000 ) ;
#36593=CARTESIAN_POINT ( 'NONE',  ( -3.306248862503413655, 500.0000000000000000, -51.64566090791306863 ) ) ;
#36606=CARTESIAN_POINT ( 'NONE',  ( 99.71998884745383407, 190.0000000000000000, 7.478223336038896996 ) ) ;
#36618=ORIENTED_EDGE ( 'NONE', *, *, #33804, .F. ) ;
#36692=CARTESIAN_POINT ( 'NONE',  ( 125.2194818923508848, 188.0000000000000000, -23.09547038499562888 ) ) ;
#36728=AXIS2_PLACEMENT_3D ( 'NONE', #61361, #13184, #7903 ) ;
#36776=FACE_OUTER_BOUND ( 'NONE', #42215, .T. ) ;
#37030=EDGE_CURVE ( 'NONE', #37226, #43800, #69468, .T. ) ;
#37107=FACE_BOUND ( 'NONE', #39399, .T. ) ;
#37113=DIRECTION ( 'NONE',  ( 1.000000000000000000, 0.000000000000000000, 0.000000000000000000 ) ) ;
#37205=ORIENTED_EDGE ( 'NONE', *, *, #41055, .F. ) ;
#37226=VERTEX_POINT ( 'NONE', #6842 ) ;
#37295=ORIENTED_EDGE ( 'NONE', *, *, #3663, .F. ) ;
#37304=ORIENTED_EDGE ( 'NONE', *, *, #68245, .F. ) ;
#37342=DIRECTION ( 'NONE',  ( -0.000000000000000000, -1.000000000000000000, 0.000000000000000000 ) ) ;
#37346=CARTESIAN_POINT ( 'NONE',  ( 99.71998884745383407, 2.000000000000001776, 7.478223336038896996 ) ) ;
#37411=VECTOR ( 'NONE', #16058, 1000.000000000000000 ) ;
#37549=CARTESIAN_POINT ( 'NONE',  ( 0.000000000000000000, 190.0000000000000000, 0.000000000000000000 ) ) ;
#37613=DIRECTION ( 'NONE',  ( -1.000000000000000000, 0.000000000000000000, 0.000000000000000000 ) ) ;
#37657=AXIS2_PLACEMENT_3D ( 'NONE', #44647, #34798, #56236 ) ;
#37707=ADVANCED_FACE ( 'NONE', ( #50378 ), #7477, .F. ) ;
#37759=CIRCLE ( 'NONE', #67076, 5.000000000000000888 ) ;
#37829=ORIENTED_EDGE ( 'NONE', *, *, #13353, .F. ) ;
#37956=DIRECTION ( 'NONE',  ( -1.000000000000000000, 0.000000000000000000, 0.000000000000000000 ) ) ;
#38002=ORIENTED_EDGE ( 'NONE', *, *, #23457, .T. ) ;
#38039=ORIENTED_EDGE ( 'NONE', *, *, #3663, .T. ) ;
#38090=DIRECTION ( 'NONE',  ( 0.000000000000000000, 0.000000000000000000, -1.000000000000000000 ) ) ;
#38150=ORIENTED_EDGE ( 'NONE', *, *, #50125, .F. ) ;
#38163=ADVANCED_FACE ( 'NONE', ( #2454 ), #45003, .F. ) ;
#38184=FACE_OUTER_BOUND ( 'NONE', #5231, .T. ) ;
#38216=ORIENTED_EDGE ( 'NONE', *, *, #4233, .F. ) ;
#38222=CARTESIAN_POINT ( 'NONE',  ( 444.9999999999999432, 225.0000000000000000, 0.000000000000000000 ) ) ;
#38240=CARTESIAN_POINT ( 'NONE',  ( 432.4999999999999432, 207.5000000000000284, 1.999999999999998224 ) ) ;
#38273=MECHANICAL_DESIGN_GEOMETRIC_PRESENTATION_REPRESENTATION('',(#65357),#11449);
#38296=CARTESIAN_POINT ( 'NONE',  ( -3.306248862503413655, 500.0000000000000000, -51.64566090791306863 ) ) ;
#38359=CARTESIAN_POINT ( 'NONE',  ( 311.0133388548732114, 190.0000000000000000, -153.4166086460792826 ) ) ;
#38382=COLOUR_RGB ( '',0.7921568627450980005, 0.8196078431372548767, 0.9333333333333333481 ) ;
#38393=CLOSED_SHELL ( 'NONE', ( #69037, #28089, #17067, #62092, #47733, #64765, #43846, #47620, #20644, #29996, #44953, #11723, #372, #66413, #33353, #34145, #27537, #955 ) ) ;
#38509=VERTEX_POINT ( 'NONE', #45272 ) ;
#38566=LINE ( 'NONE', #33310, #3787 ) ;
#38606=VERTEX_POINT ( 'NONE', #62503 ) ;
#38629=VECTOR ( 'NONE', #5353, 1000.000000000000000 ) ;
#38650=ORIENTED_EDGE ( 'NONE', *, *, #68543, .T. ) ;
#38679=DIRECTION ( 'NONE',  ( 0.000000000000000000, 0.000000000000000000, -1.000000000000000000 ) ) ;
#38797=DIRECTION ( 'NONE',  ( 0.000000000000000000, 0.000000000000000000, -1.000000000000000000 ) ) ;
#38819=CARTESIAN_POINT ( 'NONE',  ( 390.9212159716611836, 188.0000000000000000, 0.000000000000000000 ) ) ;
#38822=EDGE_CURVE ( 'NONE', #24193, #6711, #24356, .T. ) ;
#38849=AXIS2_PLACEMENT_3D ( 'NONE', #49697, #65923, #27911 ) ;
#38900=VERTEX_POINT ( 'NONE', #56346 ) ;
#38931=VECTOR ( 'NONE', #9414, 1000.000000000000000 ) ;
#38944=DIRECTION ( 'NONE',  ( 0.000000000000000000, -0.09748146057682104126, -0.9952373409613456401 ) ) ;
#38976=VERTEX_POINT ( 'NONE', #57053 ) ;
#39043=VECTOR ( 'NONE', #56282, 999.9999999999998863 ) ;
#39126=CARTESIAN_POINT ( 'NONE',  ( 149.6041652118227603, -64.71860240360767591, 1.657799476683943007 ) ) ;
#39148=EDGE_CURVE ( 'NONE', #49636, #62220, #43471, .T. ) ;
#39287=LINE ( 'NONE', #12549, #53317 ) ;
#39399=EDGE_LOOP ( 'NONE', ( #63403, #56000, #17688, #47693 ) ) ;
#39521=ORIENTED_EDGE ( 'NONE', *, *, #21135, .F. ) ;
#39672=ORIENTED_EDGE ( 'NONE', *, *, #12713, .T. ) ;
#39693=FACE_OUTER_BOUND ( 'NONE', #33001, .T. ) ;
#39726=CARTESIAN_POINT ( 'NONE',  ( 329.1355598199468204, 190.0000000000000000, -129.5087625010780812 ) ) ;
#39735=VERTEX_POINT ( 'NONE', #62633 ) ;
#39791=DIRECTION ( 'NONE',  ( 0.000000000000000000, 0.000000000000000000, 1.000000000000000000 ) ) ;
#39793=AXIS2_PLACEMENT_3D ( 'NONE', #36606, #5275, #26396 ) ;
#39849=ORIENTED_EDGE ( 'NONE', *, *, #44651, .F. ) ;
#39924=CARTESIAN_POINT ( 'NONE',  ( 444.9999999999999432, -35.00000000000000000, 2.000000000000000000 ) ) ;
#39936=LINE ( 'NONE', #61393, #55957 ) ;
#40019=EDGE_LOOP ( 'NONE', ( #54263, #61928, #63200, #37205, #25844, #46854 ) ) ;
#40057=ORIENTED_EDGE ( 'NONE', *, *, #48418, .T. ) ;
#40139=FACE_OUTER_BOUND ( 'NONE', #55336, .T. ) ;
#40248=AXIS2_PLACEMENT_3D ( 'NONE', #6385, #37342, #32080 ) ;
#40253=DIRECTION ( 'NONE',  ( 0.000000000000000000, 1.000000000000000000, 0.000000000000000000 ) ) ;
#40263=CARTESIAN_POINT ( 'NONE',  ( 311.8713128290285113, 2.000000000000001776, 346.5826552340383842 ) ) ;
#40278=FACE_OUTER_BOUND ( 'NONE', #67348, .T. ) ;
#40299=LINE ( 'NONE', #56126, #52586 ) ;
#40377=CARTESIAN_POINT ( 'NONE',  ( 427.4999999999999432, 207.5000000000000284, 1.999999999999998224 ) ) ;
#40422=CARTESIAN_POINT ( 'NONE',  ( 390.9212159716611836, 95.00000000000000000, 0.000000000000000000 ) ) ;
#40452=CARTESIAN_POINT ( 'NONE',  ( -17.50000000000000000, -17.50000000000000000, 20.00000000000000000 ) ) ;
#40518=LINE ( 'NONE', #61965, #2796 ) ;
#40520=CARTESIAN_POINT ( 'NONE',  ( 0.000000000000000000, 190.0000000000000000, 2.000000000000000000 ) ) ;
#40541=CARTESIAN_POINT ( 'NONE',  ( -22.50000000000000355, 207.5000000000000284, 0.000000000000000000 ) ) ;
#40565=EDGE_CURVE ( 'NONE', #26863, #65415, #34957, .T. ) ;
#40640=ORIENTED_EDGE ( 'NONE', *, *, #65264, .T. ) ;
#40646=VECTOR ( 'NONE', #64017, 1000.000000000000000 ) ;
#40727=ORIENTED_EDGE ( 'NONE', *, *, #13168, .T. ) ;
#40843=ORIENTED_EDGE ( 'NONE', *, *, #66760, .F. ) ;
#40944=CIRCLE ( 'NONE', #19598, 5.000000000000000888 ) ;
#41039=VECTOR ( 'NONE', #52476, 1000.000000000000000 ) ;
#41055=EDGE_CURVE ( 'NONE', #30681, #17378, #28374, .T. ) ;
#41133=DIRECTION ( 'NONE',  ( 0.000000000000000000, 1.000000000000000000, -0.000000000000000000 ) ) ;
#41139=EDGE_CURVE ( 'NONE', #25048, #54323, #7968, .T. ) ;
#41237=AXIS2_PLACEMENT_3D ( 'NONE', #58641, #31933, #6221 ) ;
#41242=VECTOR ( 'NONE', #67020, 1000.000000000000114 ) ;
#41298=PRESENTATION_STYLE_ASSIGNMENT (( #19840 ) ) ;
#41310=CARTESIAN_POINT ( 'NONE',  ( 394.5137675702981710, 500.0000000000000000, -53.65523180892861177 ) ) ;
#41354=AXIS2_PLACEMENT_3D ( 'NONE', #12361, #66200, #23618 ) ;
#41412=ORIENTED_EDGE ( 'NONE', *, *, #68531, .T. ) ;
#41426=DIRECTION ( 'NONE',  ( 0.000000000000000000, 0.000000000000000000, -1.000000000000000000 ) ) ;
#41485=AXIS2_PLACEMENT_3D ( 'NONE', #40263, #67699, #29031 ) ;
#41503=CIRCLE ( 'NONE', #57224, 298.0000000000000000 ) ;
#41519=CARTESIAN_POINT ( 'NONE',  ( 99.71998884745383407, 188.0000000000000000, 7.478223336038896996 ) ) ;
#41559=VERTEX_POINT ( 'NONE', #32449 ) ;
#41668=CARTESIAN_POINT ( 'NONE',  ( 427.4999999999999432, 207.5000000000000284, 1.999999999999998224 ) ) ;
#41725=FACE_BOUND ( 'NONE', #57086, .T. ) ;
#41735=DIRECTION ( 'NONE',  ( 0.000000000000000000, 1.000000000000000000, -0.000000000000000000 ) ) ;
#41737=CARTESIAN_POINT ( 'NONE',  ( -17.50000000000000000, 207.5000000000000284, 0.000000000000000000 ) ) ;
#41794=CARTESIAN_POINT ( 'NONE',  ( 444.9999999999999432, 225.0000000000000000, 2.000000000000000000 ) ) ;
#41960=AXIS2_PLACEMENT_3D ( 'NONE', #21340, #58281, #5510 ) ;
#41999=EDGE_CURVE ( 'NONE', #56923, #1149, #17327, .T. ) ;
#42029=CARTESIAN_POINT ( 'NONE',  ( 450.2085304802404835, 188.0000000000000000, -219.9999999999999147 ) ) ;
#42186=CIRCLE ( 'NONE', #18595, 5.000000000000000888 ) ;
#42215=EDGE_LOOP ( 'NONE', ( #63762, #63590, #7942, #50678 ) ) ;
#42355=ORIENTED_EDGE ( 'NONE', *, *, #29712, .T. ) ;
#42438=DIRECTION ( 'NONE',  ( -0.000000000000000000, 0.000000000000000000, 1.000000000000000000 ) ) ;
#42529=ORIENTED_EDGE ( 'NONE', *, *, #9097, .T. ) ;
#42575=PRESENTATION_STYLE_ASSIGNMENT (( #59773 ) ) ;
#42600=LINE ( 'NONE', #54879, #23384 ) ;
#42667=LINE ( 'NONE', #47582, #12363 ) ;
#42672=CARTESIAN_POINT ( 'NONE',  ( 173.0237957311180708, 69.97204739562489806, -91.14091141288837150 ) ) ;
#42678=VECTOR ( 'NONE', #66926, 1000.000000000000000 ) ;
#42695=DIRECTION ( 'NONE',  ( 1.000000000000000000, 0.000000000000000000, 0.000000000000000000 ) ) ;
#42736=CIRCLE ( 'NONE', #12429, 298.0000000000000000 ) ;
#42807=CARTESIAN_POINT ( 'NONE',  ( 172.9865732929135902, 70.06394889612622023, 0.000000000000000000 ) ) ;
#42872=LINE ( 'NONE', #59404, #27047 ) ;
#42902=( NAMED_UNIT ( * ) PLANE_ANGLE_UNIT ( ) SI_UNIT ( $, .RADIAN. ) );
#42942=CARTESIAN_POINT ( 'NONE',  ( 2.005731055991735623, 2.000000000000000000, 0.000000000000000000 ) ) ;
#42968=ORIENTED_EDGE ( 'NONE', *, *, #16733, .F. ) ;
#43043=VECTOR ( 'NONE', #62802, 1000.000000000000000 ) ;
#43109=DIRECTION ( 'NONE',  ( 0.000000000000000000, 0.9952373409613455291, -0.09748146057682102739 ) ) ;
#43135=EDGE_LOOP ( 'NONE', ( #65035, #20996, #6961, #57541 ) ) ;
#43156=CARTESIAN_POINT ( 'NONE',  ( 122.2516123306975402, 190.0000000000000000, -91.28179539054376335 ) ) ;
#43222=CARTESIAN_POINT ( 'NONE',  ( -17.50000000000000000, -17.50000000000000000, 0.000000000000000000 ) ) ;
#43272=ORIENTED_EDGE ( 'NONE', *, *, #9138, .F. ) ;
#43317=AXIS2_PLACEMENT_3D ( 'NONE', #16312, #15967, #6094 ) ;
#43434=VECTOR ( 'NONE', #49542, 1000.000000000000000 ) ;
#43444=CARTESIAN_POINT ( 'NONE',  ( 311.9732115134679020, 2.000000000000000000, -151.4173343409194672 ) ) ;
#43448=ORIENTED_EDGE ( 'NONE', *, *, #61245, .F. ) ;
#43471=LINE ( 'NONE', #49089, #62073 ) ;
#43513=EDGE_LOOP ( 'NONE', ( #54301, #28963, #14899, #33751 ) ) ;
#43581=CARTESIAN_POINT ( 'NONE',  ( 427.4999999999999432, 207.5000000000000284, 20.00000000000000000 ) ) ;
#43593=ORIENTED_EDGE ( 'NONE', *, *, #11182, .T. ) ;
#43606=ORIENTED_EDGE ( 'NONE', *, *, #38822, .F. ) ;
#43693=ORIENTED_EDGE ( 'NONE', *, *, #28029, .T. ) ;
#43736=AXIS2_PLACEMENT_3D ( 'NONE', #40452, #25331, #14066 ) ;
#43779=ORIENTED_EDGE ( 'NONE', *, *, #26236, .F. ) ;
#43800=VERTEX_POINT ( 'NONE', #51970 ) ;
#43804=EDGE_CURVE ( 'NONE', #38606, #5953, #14064, .T. ) ;
#43814=ORIENTED_EDGE ( 'NONE', *, *, #45983, .T. ) ;
#43823=DIRECTION ( 'NONE',  ( -0.000000000000000000, -1.000000000000000000, -0.000000000000000000 ) ) ;
#43846=ADVANCED_FACE ( 'NONE', ( #24905 ), #62536, .F. ) ;
#43904=DIRECTION ( 'NONE',  ( -0.000000000000000000, -1.000000000000000000, -0.000000000000000000 ) ) ;
#43913=CARTESIAN_POINT ( 'NONE',  ( 259.2042601260359334, 188.0000000000000000, 7.478223336038896996 ) ) ;
#43934=FACE_OUTER_BOUND ( 'NONE', #22291, .T. ) ;
#43935=VERTEX_POINT ( 'NONE', #3328 ) ;
#44112=VERTEX_POINT ( 'NONE', #23334 ) ;
#44158=CARTESIAN_POINT ( 'NONE',  ( 544.6745185807129701, 190.0000000000000000, 34.73878747406611467 ) ) ;
#44185=DIRECTION ( 'NONE',  ( 0.000000000000000000, -0.000000000000000000, 1.000000000000000000 ) ) ;
#44251=ORIENTED_EDGE ( 'NONE', *, *, #7799, .F. ) ;
#44265=VERTEX_POINT ( 'NONE', #38359 ) ;
#44308=DIRECTION ( 'NONE',  ( -0.9174381082928754205, 0.3978785209734126416, 0.000000000000000000 ) ) ;
#44558=DIRECTION ( 'NONE',  ( 0.000000000000000000, 0.000000000000000000, 1.000000000000000000 ) ) ;
#44597=LINE ( 'NONE', #17870, #32958 ) ;
#44630=DIRECTION ( 'NONE',  ( 0.000000000000000000, 1.000000000000000000, -0.000000000000000000 ) ) ;
#44647=CARTESIAN_POINT ( 'NONE',  ( 311.8713128290285113, 0.000000000000000000, 346.5826552340383842 ) ) ;
#44651=EDGE_CURVE ( 'NONE', #9244, #14749, #51196, .T. ) ;
#44701=CARTESIAN_POINT ( 'NONE',  ( 444.9999999999999432, -35.00000000000000000, 2.000000000000000000 ) ) ;
#44731=DIRECTION ( 'NONE',  ( 0.000000000000000000, -1.000000000000000000, 0.000000000000000000 ) ) ;
#44763=DIRECTION ( 'NONE',  ( 0.000000000000000000, 0.000000000000000000, -1.000000000000000000 ) ) ;
#44819=DIRECTION ( 'NONE',  ( -0.000000000000000000, 0.001173758924898823768, 0.9999993111447559313 ) ) ;
#44890=ORIENTED_EDGE ( 'NONE', *, *, #65264, .F. ) ;
#44903=FACE_OUTER_BOUND ( 'NONE', #54832, .T. ) ;
#44934=EDGE_CURVE ( 'NONE', #22712, #1594, #16652, .T. ) ;
#44953=ADVANCED_FACE ( 'NONE', ( #54633 ), #16994, .T. ) ;
#45003=PLANE ( 'NONE',  #55290 ) ;
#45100=ORIENTED_EDGE ( 'NONE', *, *, #7799, .T. ) ;
#45105=CARTESIAN_POINT ( 'NONE',  ( 410.0000000000000000, 190.0000000000000000, 2.000000000000000000 ) ) ;
#45109=PRODUCT ( 'cover', 'cover', '', ( #59258 ) ) ;
#45178=CYLINDRICAL_SURFACE ( 'NONE', #36728, 99.99999999999994316 ) ;
#45185=EDGE_CURVE ( 'NONE', #37226, #11952, #20463, .T. ) ;
#45198=VERTEX_POINT ( 'NONE', #40541 ) ;
#45212=DIRECTION ( 'NONE',  ( 1.000000000000000000, 0.000000000000000000, 0.000000000000000000 ) ) ;
#45215=AXIS2_PLACEMENT_3D ( 'NONE', #28181, #11652, #10965 ) ;
#45237=CARTESIAN_POINT ( 'NONE',  ( 47.74291447196797833, 188.0000000000000000, -75.60236247897087480 ) ) ;
#45272=CARTESIAN_POINT ( 'NONE',  ( 450.2085304802404835, 190.0000000000000000, -219.9999999999999147 ) ) ;
#45310=DIRECTION ( 'NONE',  ( 0.000000000000000000, 0.000000000000000000, -1.000000000000000000 ) ) ;
#45390=FACE_OUTER_BOUND ( 'NONE', #19815, .T. ) ;
#45567=CIRCLE ( 'NONE', #11813, 5.000000000000004441 ) ;
#45577=LINE ( 'NONE', #67395, #43043 ) ;
#45622=AXIS2_PLACEMENT_3D ( 'NONE', #3802, #15394, #46016 ) ;
#45626=VECTOR ( 'NONE', #48559, 1000.000000000000000 ) ;
#45633=CARTESIAN_POINT ( 'NONE',  ( 0.000000000000000000, 0.000000000000000000, 0.000000000000000000 ) ) ;
#45710=CARTESIAN_POINT ( 'NONE',  ( 151.3797687388446889, -65.65103187525450323, 0.000000000000000000 ) ) ;
#45715=AXIS2_PLACEMENT_3D ( 'NONE', #45877, #52531, #2976 ) ;
#45743=PLANE ( 'NONE',  #32852 ) ;
#45762=EDGE_CURVE ( 'NONE', #25024, #61751, #26566, .T. ) ;
#45765=CARTESIAN_POINT ( 'NONE',  ( 450.2085304802404266, 190.0000000000000000, -250.0000000000000000 ) ) ;
#45772=ORIENTED_EDGE ( 'NONE', *, *, #50653, .F. ) ;
#45877=CARTESIAN_POINT ( 'NONE',  ( 99.71998884745383407, 0.000000000000000000, 7.478223336038896996 ) ) ;
#45963=DIRECTION ( 'NONE',  ( 1.000000000000000000, 0.000000000000000000, 0.000000000000000000 ) ) ;
#45983=EDGE_CURVE ( 'NONE', #27607, #60636, #57603, .T. ) ;
#45991=DIRECTION ( 'NONE',  ( 0.000000000000000000, 1.000000000000000000, -0.000000000000000000 ) ) ;
#46016=DIRECTION ( 'NONE',  ( -1.000000000000000000, 0.000000000000000000, 0.000000000000000000 ) ) ;
#46023=ORIENTED_EDGE ( 'NONE', *, *, #28231, .T. ) ;
#46027=ORIENTED_EDGE ( 'NONE', *, *, #62367, .F. ) ;
#46038=ORIENTED_EDGE ( 'NONE', *, *, #13125, .F. ) ;
#46162=DIRECTION ( 'NONE',  ( -0.3738650651659383151, 0.9230658208099267181, -0.09041240789275074852 ) ) ;
#46174=ORIENTED_EDGE ( 'NONE', *, *, #50125, .T. ) ;
#46200=EDGE_CURVE ( 'NONE', #3462, #38900, #3972, .T. ) ;
#46296=CARTESIAN_POINT ( 'NONE',  ( 0.000000000000000000, 0.000000000000000000, 0.000000000000000000 ) ) ;
#46327=DIRECTION ( 'NONE',  ( 0.000000000000000000, 0.000000000000000000, -1.000000000000000000 ) ) ;
#46370=VECTOR ( 'NONE', #5102, 1000.000000000000000 ) ;
#46374=VECTOR ( 'NONE', #7940, 1000.000000000000000 ) ;
#46408=VECTOR ( 'NONE', #49503, 1000.000000000000000 ) ;
#46523=CYLINDRICAL_SURFACE ( 'NONE', #68064, 5.000000000000000888 ) ;
#46587=ADVANCED_FACE ( 'NONE', ( #34870 ), #18330, .F. ) ;
#46628=( LENGTH_UNIT ( ) NAMED_UNIT ( * ) SI_UNIT ( .MILLI., .METRE. ) );
#46748=VECTOR ( 'NONE', #46162, 1000.000000000000000 ) ;
#46749=DIRECTION ( 'NONE',  ( 0.000000000000000000, 0.000000000000000000, -1.000000000000000000 ) ) ;
#46854=ORIENTED_EDGE ( 'NONE', *, *, #36518, .T. ) ;
#46856=CIRCLE ( 'NONE', #15437, 99.99999999999994316 ) ;
#46886=DIRECTION ( 'NONE',  ( 0.000000000000000000, 0.000000000000000000, -1.000000000000000000 ) ) ;
#46962=CYLINDRICAL_SURFACE ( 'NONE', #34885, 298.0000000000000000 ) ;
#46998=DIRECTION ( 'NONE',  ( 0.000000000000000000, 0.000000000000000000, -1.000000000000000000 ) ) ;
#47040=CARTESIAN_POINT ( 'NONE',  ( 544.6745185807129701, 2.000000000000001776, 34.73878747406611467 ) ) ;
#47309=CARTESIAN_POINT ( 'NONE',  ( 396.6937511374966334, 500.0000000000000000, -91.64566090791306863 ) ) ;
#47339=ORIENTED_EDGE ( 'NONE', *, *, #54944, .T. ) ;
#47422=CIRCLE ( 'NONE', #9273, 5.000000000000000888 ) ;
#47441=DIRECTION ( 'NONE',  ( -0.000000000000000000, -1.000000000000000000, -0.000000000000000000 ) ) ;
#47469=DIRECTION ( 'NONE',  ( 0.000000000000000000, 0.000000000000000000, -1.000000000000000000 ) ) ;
#47473=ORIENTED_EDGE ( 'NONE', *, *, #28029, .F. ) ;
#47487=DIRECTION ( 'NONE',  ( -0.000000000000000000, -0.000000000000000000, -1.000000000000000000 ) ) ;
#47498=CIRCLE ( 'NONE', #64377, 5.000000000000004441 ) ;
#47573=APPLICATION_CONTEXT ( 'automotive_design' ) ;
#47582=CARTESIAN_POINT ( 'NONE',  ( 149.5059104800819796, -64.94516058774519252, -90.98255102680806772 ) ) ;
#47584=ORIENTED_EDGE ( 'NONE', *, *, #45185, .T. ) ;
#47620=ADVANCED_FACE ( 'NONE', ( #15827 ), #26048, .F. ) ;
#47626=ORIENTED_EDGE ( 'NONE', *, *, #58189, .T. ) ;
#47693=ORIENTED_EDGE ( 'NONE', *, *, #28231, .F. ) ;
#47733=ADVANCED_FACE ( 'NONE', ( #63500, #9341, #69456, #20579, #36776, #37107 ), #14283, .T. ) ;
#47755=CIRCLE ( 'NONE', #37657, 500.0000000000000000 ) ;
#47808=CARTESIAN_POINT ( 'NONE',  ( 0.000000000000000000, -0.1068809833119260672, -91.05865558859387932 ) ) ;
#47852=VECTOR ( 'NONE', #32467, 1000.000000000000114 ) ;
#48021=DIRECTION ( 'NONE',  ( 1.000000000000000000, 0.000000000000000000, 0.000000000000000000 ) ) ;
#48037=DIRECTION ( 'NONE',  ( 0.000000000000000000, -0.09748146057682104126, -0.9952373409613456401 ) ) ;
#48066=ORIENTED_EDGE ( 'NONE', *, *, #13125, .T. ) ;
#48121=EDGE_CURVE ( 'NONE', #1594, #62220, #12032, .T. ) ;
#48210=CARTESIAN_POINT ( 'NONE',  ( 450.2085304802404266, 190.0000000000000000, -250.0000000000000000 ) ) ;
#48315=ORIENTED_EDGE ( 'NONE', *, *, #62281, .F. ) ;
#48418=EDGE_CURVE ( 'NONE', #16361, #68856, #50976, .T. ) ;
#48450=DIRECTION ( 'NONE',  ( 1.000000000000000000, 0.000000000000000000, 0.000000000000000000 ) ) ;
#48480=DIRECTION ( 'NONE',  ( -1.000000000000000000, 0.000000000000000000, 0.000000000000000000 ) ) ;
#48559=DIRECTION ( 'NONE',  ( 0.000000000000000000, 0.000000000000000000, 1.000000000000000000 ) ) ;
#48597=VECTOR ( 'NONE', #1554, 1000.000000000000000 ) ;
#48623=EDGE_CURVE ( 'NONE', #25048, #8863, #23418, .T. ) ;
#48652=CARTESIAN_POINT ( 'NONE',  ( -22.50000000000000355, -17.50000000000000000, 0.000000000000000000 ) ) ;
#48690=VECTOR ( 'NONE', #59399, 1000.000000000000000 ) ;
#48744=CYLINDRICAL_SURFACE ( 'NONE', #19072, 300.0000000000000000 ) ;
#48836=CIRCLE ( 'NONE', #58945, 300.0000000000000000 ) ;
#48950=VECTOR ( 'NONE', #28972, 1000.000000000000000 ) ;
#49048=EDGE_CURVE ( 'NONE', #44112, #17378, #5418, .T. ) ;
#49084=LINE ( 'NONE', #33640, #31764 ) ;
#49089=CARTESIAN_POINT ( 'NONE',  ( 0.000000000000000000, 500.0000000000000000, -53.65523180892861177 ) ) ;
#49152=DIRECTION ( 'NONE',  ( -0.000000000000000000, -0.000000000000000000, -1.000000000000000000 ) ) ;
#49250=CARTESIAN_POINT ( 'NONE',  ( 173.3767798452622912, 69.10053625052562154, -11.44951126442670386 ) ) ;
#49309=DIRECTION ( 'NONE',  ( 0.000000000000000000, 0.000000000000000000, -1.000000000000000000 ) ) ;
#49320=DIRECTION ( 'NONE',  ( -0.000000000000000000, -1.000000000000000000, 0.000000000000000000 ) ) ;
#49367=EDGE_LOOP ( 'NONE', ( #37295, #31312, #21244, #14392 ) ) ;
#49412=CARTESIAN_POINT ( 'NONE',  ( 444.9999999999999432, 225.0000000000000000, 2.000000000000000000 ) ) ;
#49464=DIRECTION ( 'NONE',  ( 0.000000000000000000, 0.9952373409613455291, -0.09748146057682102739 ) ) ;
#49475=CARTESIAN_POINT ( 'NONE',  ( -12.50000000000000000, -17.50000000000000000, 0.000000000000000000 ) ) ;
#49494=DIRECTION ( 'NONE',  ( -1.000000000000000000, 0.000000000000000000, 0.000000000000000000 ) ) ;
#49500=ORIENTED_EDGE ( 'NONE', *, *, #18750, .T. ) ;
#49503=DIRECTION ( 'NONE',  ( -0.000000000000000000, -0.000000000000000000, 1.000000000000000000 ) ) ;
#49530=ORIENTED_EDGE ( 'NONE', *, *, #72, .T. ) ;
#49542=DIRECTION ( 'NONE',  ( -0.000000000000000000, -1.000000000000000000, -0.000000000000000000 ) ) ;
#49636=VERTEX_POINT ( 'NONE', #18281 ) ;
#49675=DIRECTION ( 'NONE',  ( 0.000000000000000000, -1.000000000000000000, 0.000000000000000000 ) ) ;
#49697=CARTESIAN_POINT ( 'NONE',  ( 171.1328495613745417, 69.31314377685163208, 0.000000000000000000 ) ) ;
#49739=LINE ( 'NONE', #56085, #34326 ) ;
#49775=ORIENTED_EDGE ( 'NONE', *, *, #53021, .F. ) ;
#49779=ORIENTED_EDGE ( 'NONE', *, *, #11317, .T. ) ;
#49863=CARTESIAN_POINT ( 'NONE',  ( 122.2516123306975402, 190.0000000000000000, -21.28179539054375624 ) ) ;
#49897=LINE ( 'NONE', #29150, #57287 ) ;
#49929=CARTESIAN_POINT ( 'NONE',  ( 262.2516123306975260, 190.0000000000000000, -21.28179539054375624 ) ) ;
#50057=VERTEX_POINT ( 'NONE', #3749 ) ;
#50086=VECTOR ( 'NONE', #63027, 1000.000000000000000 ) ;
#50125=EDGE_CURVE ( 'NONE', #38976, #6944, #16604, .T. ) ;
#50216=ORIENTED_EDGE ( 'NONE', *, *, #67855, .F. ) ;
#50257=CYLINDRICAL_SURFACE ( 'NONE', #57954, 5.000000000000000888 ) ;
#50378=FACE_OUTER_BOUND ( 'NONE', #43513, .T. ) ;
#50385=ADVANCED_FACE ( 'NONE', ( #3665 ), #24448, .F. ) ;
#50461=CARTESIAN_POINT ( 'NONE',  ( 329.1355598199468204, 0.000000000000000000, -129.5087625010780812 ) ) ;
#50485=CARTESIAN_POINT ( 'NONE',  ( -12.50000000000000000, 207.5000000000000284, 0.000000000000000000 ) ) ;
#50502=CYLINDRICAL_SURFACE ( 'NONE', #35138, 5.000000000000004441 ) ;
#50504=ORIENTED_EDGE ( 'NONE', *, *, #41055, .T. ) ;
#50530=CARTESIAN_POINT ( 'NONE',  ( 0.000000000000000000, 0.000000000000000000, 0.000000000000000000 ) ) ;
#50599=CARTESIAN_POINT ( 'NONE',  ( -17.50000000000000000, 207.5000000000000284, 20.00000000000000000 ) ) ;
#50614=CYLINDRICAL_SURFACE ( 'NONE', #62588, 299.9999999999999432 ) ;
#50653=EDGE_CURVE ( 'NONE', #32859, #56923, #28773, .T. ) ;
#50678=ORIENTED_EDGE ( 'NONE', *, *, #23089, .T. ) ;
#50773=ORIENTED_EDGE ( 'NONE', *, *, #65368, .F. ) ;
#50870=CARTESIAN_POINT ( 'NONE',  ( 0.000000000000000000, -0.4541622202827808596, -4.636770908075737552 ) ) ;
#50879=VERTEX_POINT ( 'NONE', #50485 ) ;
#50895=DIRECTION ( 'NONE',  ( -0.000000000000000000, -1.000000000000000000, -0.000000000000000000 ) ) ;
#50976=LINE ( 'NONE', #34809, #51483 ) ;
#51004=ORIENTED_EDGE ( 'NONE', *, *, #48121, .T. ) ;
#51055=CARTESIAN_POINT ( 'NONE',  ( 444.9999999999999432, 225.0000000000000000, 2.000000000000000000 ) ) ;
#51196=LINE ( 'NONE', #61395, #20840 ) ;
#51226=( NAMED_UNIT ( * ) SI_UNIT ( $, .STERADIAN. ) SOLID_ANGLE_UNIT ( ) );
#51240=AXIS2_PLACEMENT_3D ( 'NONE', #64694, #44630, #1368 ) ;
#51253=FACE_BOUND ( 'NONE', #36359, .T. ) ;
#51316=FACE_OUTER_BOUND ( 'NONE', #19960, .T. ) ;
#51318=DIRECTION ( 'NONE',  ( -0.000000000000000000, -0.000000000000000000, -1.000000000000000000 ) ) ;
#51331=CARTESIAN_POINT ( 'NONE',  ( 149.5448925222589196, -64.85527483330767495, 0.000000000000000000 ) ) ;
#51342=AXIS2_PLACEMENT_3D ( 'NONE', #41794, #30896, #4164 ) ;
#51440=CARTESIAN_POINT ( 'NONE',  ( 410.0000000000000000, 0.000000000000000000, 0.000000000000000000 ) ) ;
#51483=VECTOR ( 'NONE', #56247, 1000.000000000000114 ) ;
#51492=EDGE_CURVE ( 'NONE', #43935, #59387, #54884, .T. ) ;
#51584=ORIENTED_EDGE ( 'NONE', *, *, #8106, .T. ) ;
#51626=ORIENTED_EDGE ( 'NONE', *, *, #26594, .F. ) ;
#51633=COLOUR_RGB ( '',0.7921568627450980005, 0.8196078431372548767, 0.9333333333333333481 ) ;
#51660=EDGE_CURVE ( 'NONE', #38509, #14449, #68238, .T. ) ;
#51668=AXIS2_PLACEMENT_3D ( 'NONE', #22463, #43904, #17173 ) ;
#51696=DIRECTION ( 'NONE',  ( 0.000000000000000000, 1.000000000000000000, -0.000000000000000000 ) ) ;
#51712=ORIENTED_EDGE ( 'NONE', *, *, #57557, .F. ) ;
#51728=FACE_OUTER_BOUND ( 'NONE', #27260, .T. ) ;
#51834=EDGE_LOOP ( 'NONE', ( #23595, #58504 ) ) ;
#51874=DIRECTION ( 'NONE',  ( 1.000000000000000000, 0.000000000000000000, 0.000000000000000000 ) ) ;
#51970=CARTESIAN_POINT ( 'NONE',  ( 262.2516123306975260, 190.0000000000000000, -21.28179539054375624 ) ) ;
#52044=VECTOR ( 'NONE', #1453, 1000.000000000000000 ) ;
#52071=DIRECTION ( 'NONE',  ( 0.000000000000000000, -1.000000000000000000, 0.000000000000000000 ) ) ;
#52208=EDGE_LOOP ( 'NONE', ( #57021, #69455, #1518, #55989 ) ) ;
#52332=FACE_OUTER_BOUND ( 'NONE', #63013, .T. ) ;
#52419=PLANE ( 'NONE',  #35626 ) ;
#52426=VERTEX_POINT ( 'NONE', #33386 ) ;
#52476=DIRECTION ( 'NONE',  ( 0.000000000000000000, 0.000000000000000000, -1.000000000000000000 ) ) ;
#52491=AXIS2_PLACEMENT_3D ( 'NONE', #41668, #30425, #51874 ) ;
#52525=CIRCLE ( 'NONE', #22193, 299.9999999999999432 ) ;
#52531=DIRECTION ( 'NONE',  ( 0.000000000000000000, -1.000000000000000000, 0.000000000000000000 ) ) ;
#52586=VECTOR ( 'NONE', #28712, 1000.000000000000000 ) ;
#52651=CARTESIAN_POINT ( 'NONE',  ( 99.71998884745383407, 2.000000000000000000, 0.000000000000000000 ) ) ;
#52674=ORIENTED_EDGE ( 'NONE', *, *, #66788, .T. ) ;
#52678=CARTESIAN_POINT ( 'NONE',  ( 410.0000000000000000, 190.0000000000000000, -90.00000000000000000 ) ) ;
#52689=DIRECTION ( 'NONE',  ( 1.000000000000000000, 0.000000000000000000, 0.000000000000000000 ) ) ;
#52732=DIRECTION ( 'NONE',  ( 0.000000000000000000, 0.000000000000000000, -1.000000000000000000 ) ) ;
#52743=DIRECTION ( 'NONE',  ( -0.000000000000000000, -1.000000000000000000, -0.000000000000000000 ) ) ;
#52833=CARTESIAN_POINT ( 'NONE',  ( 0.000000000000000000, 0.000000000000000000, 2.000000000000000000 ) ) ;
#52871=ADVANCED_FACE ( 'NONE', ( #22219 ), #765, .F. ) ;
#52904=ORIENTED_EDGE ( 'NONE', *, *, #1100, .T. ) ;
#53021=EDGE_CURVE ( 'NONE', #61986, #55566, #14706, .T. ) ;
#53112=VERTEX_POINT ( 'NONE', #35828 ) ;
#53113=ORIENTED_EDGE ( 'NONE', *, *, #43804, .F. ) ;
#53237=CARTESIAN_POINT ( 'NONE',  ( 99.71998884745383407, 188.0000000000000000, -23.09547038499562888 ) ) ;
#53317=VECTOR ( 'NONE', #61083, 1000.000000000000000 ) ;
#53449=EDGE_LOOP ( 'NONE', ( #44890, #47473, #51004, #27401, #32389 ) ) ;
#53736=ORIENTED_EDGE ( 'NONE', *, *, #9097, .F. ) ;
#53831=DIRECTION ( 'NONE',  ( -0.000000000000000000, -1.000000000000000000, -0.000000000000000000 ) ) ;
#53859=STYLED_ITEM ( 'NONE', ( #41298 ), #65110 ) ;
#53939=DIRECTION ( 'NONE',  ( 1.000000000000000000, 0.000000000000000000, 0.000000000000000000 ) ) ;
#54226=DIRECTION ( 'NONE',  ( -0.3978785209734125861, -0.9174381082928753095, 0.000000000000000000 ) ) ;
#54229=VERTEX_POINT ( 'NONE', #38240 ) ;
#54263=ORIENTED_EDGE ( 'NONE', *, *, #55811, .T. ) ;
#54301=ORIENTED_EDGE ( 'NONE', *, *, #29375, .T. ) ;
#54323=VERTEX_POINT ( 'NONE', #49475 ) ;
#54424=PLANE ( 'NONE',  #55308 ) ;
#54481=AXIS2_PLACEMENT_3D ( 'NONE', #32559, #41735, #32220 ) ;
#54501=DIRECTION ( 'NONE',  ( 1.000000000000000000, 0.000000000000000000, 0.000000000000000000 ) ) ;
#54524=VECTOR ( 'NONE', #57498, 1000.000000000000000 ) ;
#54613=ADVANCED_FACE ( 'NONE', ( #6504 ), #34290, .F. ) ;
#54633=FACE_OUTER_BOUND ( 'NONE', #66208, .T. ) ;
#54688=ORIENTED_EDGE ( 'NONE', *, *, #1850, .F. ) ;
#54739=DIRECTION ( 'NONE',  ( 0.000000000000000000, 1.000000000000000000, 0.000000000000000000 ) ) ;
#54803=ORIENTED_EDGE ( 'NONE', *, *, #62281, .T. ) ;
#54832=EDGE_LOOP ( 'NONE', ( #62255, #67781, #39672, #9977 ) ) ;
#54858=LINE ( 'NONE', #22168, #17231 ) ;
#54879=CARTESIAN_POINT ( 'NONE',  ( 422.4999999999999432, 207.5000000000000284, 20.00000000000000000 ) ) ;
#54884=LINE ( 'NONE', #6707, #18165 ) ;
#54924=CIRCLE ( 'NONE', #41485, 498.0000000000000000 ) ;
#54944=EDGE_CURVE ( 'NONE', #44265, #43935, #4885, .T. ) ;
#54994=LINE ( 'NONE', #1910, #18053 ) ;
#55090=CARTESIAN_POINT ( 'NONE',  ( 2.005731055991735623, 188.0000000000000000, 0.000000000000000000 ) ) ;
#55168=EDGE_CURVE ( 'NONE', #1149, #31022, #54858, .T. ) ;
#55181=DIRECTION ( 'NONE',  ( -0.000000000000000000, -1.000000000000000000, -0.000000000000000000 ) ) ;
#55290=AXIS2_PLACEMENT_3D ( 'NONE', #45710, #44308, #55561 ) ;
#55308=AXIS2_PLACEMENT_3D ( 'NONE', #11878, #49494, #60420 ) ;
#55336=EDGE_LOOP ( 'NONE', ( #25759, #3323, #6862, #13804 ) ) ;
#55362=LINE ( 'NONE', #28281, #48597 ) ;
#55378=DIRECTION ( 'NONE',  ( -1.000000000000000000, 0.000000000000000000, 0.000000000000000000 ) ) ;
#55383=ORIENTED_EDGE ( 'NONE', *, *, #29638, .T. ) ;
#55528=CARTESIAN_POINT ( 'NONE',  ( 450.2085304802404266, 188.0000000000000000, -247.8920266495912870 ) ) ;
#55561=DIRECTION ( 'NONE',  ( -0.3978785209734125861, -0.9174381082928753095, 0.000000000000000000 ) ) ;
#55566=VERTEX_POINT ( 'NONE', #19846 ) ;
#55608=ORIENTED_EDGE ( 'NONE', *, *, #26236, .T. ) ;
#55611=ORIENTED_EDGE ( 'NONE', *, *, #33006, .T. ) ;
#55637=ORIENTED_EDGE ( 'NONE', *, *, #48418, .F. ) ;
#55704=DIRECTION ( 'NONE',  ( -0.000000000000000000, -1.000000000000000000, -0.000000000000000000 ) ) ;
#55752=VECTOR ( 'NONE', #18593, 1000.000000000000000 ) ;
#55765=DIRECTION ( 'NONE',  ( -1.000000000000000000, 0.000000000000000000, 0.000000000000000000 ) ) ;
#55811=EDGE_CURVE ( 'NONE', #11580, #25024, #65611, .T. ) ;
#55909=ORIENTED_EDGE ( 'NONE', *, *, #28424, .F. ) ;
#55951=EDGE_LOOP ( 'NONE', ( #11442, #51584, #57888, #43693 ) ) ;
#55957=VECTOR ( 'NONE', #7931, 1000.000000000000000 ) ;
#55981=EDGE_CURVE ( 'NONE', #61751, #19234, #40518, .T. ) ;
#55982=PLANE ( 'NONE',  #25341 ) ;
#55989=ORIENTED_EDGE ( 'NONE', *, *, #30337, .T. ) ;
#56000=ORIENTED_EDGE ( 'NONE', *, *, #45983, .F. ) ;
#56008=CARTESIAN_POINT ( 'NONE',  ( 410.0000000000000000, 0.000000000000000000, 2.000000000000000000 ) ) ;
#56055=DIRECTION ( 'NONE',  ( 0.000000000000000000, 0.000000000000000000, -1.000000000000000000 ) ) ;
#56085=CARTESIAN_POINT ( 'NONE',  ( 444.9999999999999432, -35.00000000000000000, 0.000000000000000000 ) ) ;
#56126=CARTESIAN_POINT ( 'NONE',  ( 324.1677456657756125, 188.0000000000000000, -123.1183350412580779 ) ) ;
#56197=CARTESIAN_POINT ( 'NONE',  ( 544.6745185807129701, 188.0000000000000000, 34.73878747406611467 ) ) ;
#56236=DIRECTION ( 'NONE',  ( 0.000000000000000000, 0.000000000000000000, -1.000000000000000000 ) ) ;
#56247=DIRECTION ( 'NONE',  ( -0.3754023374827052950, 0.9268613172740186590, -0.001087912492708085609 ) ) ;
#56259=VECTOR ( 'NONE', #17021, 1000.000000000000000 ) ;
#56262=DIRECTION ( 'NONE',  ( -0.000000000000000000, -0.000000000000000000, -1.000000000000000000 ) ) ;
#56272=DIRECTION ( 'NONE',  ( 0.000000000000000000, 0.000000000000000000, -1.000000000000000000 ) ) ;
#56282=DIRECTION ( 'NONE',  ( 0.3978782902816504485, 0.9174375763581197329, -0.001076851285082543923 ) ) ;
#56346=CARTESIAN_POINT ( 'NONE',  ( 450.2085304802404266, 2.000000000000000000, -247.8920266495912870 ) ) ;
#56395=FACE_OUTER_BOUND ( 'NONE', #28031, .T. ) ;
#56490=CARTESIAN_POINT ( 'NONE',  ( 450.2085304802404266, 188.0000000000000000, -247.8920266495912870 ) ) ;
#56498=VECTOR ( 'NONE', #60732, 1000.000000000000000 ) ;
#56510=FACE_BOUND ( 'NONE', #23428, .T. ) ;
#56538=EDGE_CURVE ( 'NONE', #39735, #58197, #34285, .T. ) ;
#56615=VERTEX_POINT ( 'NONE', #6869 ) ;
#56652=CARTESIAN_POINT ( 'NONE',  ( 311.0133388548732114, 0.000000000000000000, -153.4166086460792826 ) ) ;
#56733=CARTESIAN_POINT ( 'NONE',  ( -17.50000000000000000, -17.50000000000000000, 1.999999999999998224 ) ) ;
#56851=( NAMED_UNIT ( * ) PLANE_ANGLE_UNIT ( ) SI_UNIT ( $, .RADIAN. ) );
#56923=VERTEX_POINT ( 'NONE', #22270 ) ;
#56994=CARTESIAN_POINT ( 'NONE',  ( 422.4999999999999432, -17.50000000000000000, 1.999999999999998224 ) ) ;
#57012=DIRECTION ( 'NONE',  ( -0.000000000000000000, -1.000000000000000000, -0.000000000000000000 ) ) ;
#57021=ORIENTED_EDGE ( 'NONE', *, *, #26622, .F. ) ;
#57053=CARTESIAN_POINT ( 'NONE',  ( -12.50000000000000000, 207.5000000000000284, 1.999999999999998224 ) ) ;
#57056=CARTESIAN_POINT ( 'NONE',  ( 394.5137675702981710, 500.0000000000000000, 0.000000000000000000 ) ) ;
#57086=EDGE_LOOP ( 'NONE', ( #57280, #67806 ) ) ;
#57135=FILL_AREA_STYLE ('',( #35682 ) ) ;
#57204=EDGE_LOOP ( 'NONE', ( #51626, #3923, #4565, #20973, #560, #13102, #5500, #64378 ) ) ;
#57209=CARTESIAN_POINT ( 'NONE',  ( 444.9999999999999432, -35.00000000000000000, 0.000000000000000000 ) ) ;
#57216=PLANE ( 'NONE',  #58339 ) ;
#57224=AXIS2_PLACEMENT_3D ( 'NONE', #56197, #45991, #46327 ) ;
#57227=DIRECTION ( 'NONE',  ( 1.000000000000000000, 0.000000000000000000, 0.000000000000000000 ) ) ;
#57256=DIRECTION ( 'NONE',  ( -0.000000000000000000, 0.000000000000000000, -1.000000000000000000 ) ) ;
#57280=ORIENTED_EDGE ( 'NONE', *, *, #627, .F. ) ;
#57287=VECTOR ( 'NONE', #23875, 1000.000000000000000 ) ;
#57392=CARTESIAN_POINT ( 'NONE',  ( 394.5137675702982847, 500.0000000000001137, -91.64566090791306863 ) ) ;
#57403=CARTESIAN_POINT ( 'NONE',  ( 432.4999999999999432, -17.50000000000000000, 20.00000000000000000 ) ) ;
#57436=CARTESIAN_POINT ( 'NONE',  ( 450.2085304802404266, 2.000000000000000000, 7.478223336038896996 ) ) ;
#57498=DIRECTION ( 'NONE',  ( -0.000000000000000000, -1.000000000000000000, -0.000000000000000000 ) ) ;
#57501=ORIENTED_EDGE ( 'NONE', *, *, #62745, .F. ) ;
#57541=ORIENTED_EDGE ( 'NONE', *, *, #2634, .F. ) ;
#57557=EDGE_CURVE ( 'NONE', #59365, #14479, #68401, .T. ) ;
#57603=LINE ( 'NONE', #8381, #38931 ) ;
#57610=EDGE_LOOP ( 'NONE', ( #31323, #16334, #10773, #67886, #55383, #34107, #47339 ) ) ;
#57630=PLANE ( 'NONE',  #51342 ) ;
#57691=FACE_OUTER_BOUND ( 'NONE', #66161, .T. ) ;
#57699=CARTESIAN_POINT ( 'NONE',  ( 450.2085304802404266, 190.0000000000000000, -250.0000000000000000 ) ) ;
#57767=AXIS2_PLACEMENT_3D ( 'NONE', #37346, #58802, #46886 ) ;
#57842=ORIENTED_EDGE ( 'NONE', *, *, #16598, .T. ) ;
#57888=ORIENTED_EDGE ( 'NONE', *, *, #44934, .T. ) ;
#57932=LINE ( 'NONE', #62164, #33647 ) ;
#57954=AXIS2_PLACEMENT_3D ( 'NONE', #50599, #61158, #2080 ) ;
#58019=CARTESIAN_POINT ( 'NONE',  ( 450.2085304802404835, 190.0000000000000000, -219.9999999999999147 ) ) ;
#58058=CIRCLE ( 'NONE', #41237, 5.000000000000004441 ) ;
#58101=PRODUCT_DEFINITION ( 'UNKNOWN', '', #17593, #5692 ) ;
#58189=EDGE_CURVE ( 'NONE', #28423, #15622, #31708, .T. ) ;
#58195=CARTESIAN_POINT ( 'NONE',  ( -35.00000000000000000, -35.00000000000000000, 0.000000000000000000 ) ) ;
#58197=VERTEX_POINT ( 'NONE', #25416 ) ;
#58281=DIRECTION ( 'NONE',  ( 0.000000000000000000, -1.000000000000000000, 0.000000000000000000 ) ) ;
#58339=AXIS2_PLACEMENT_3D ( 'NONE', #46296, #30477, #45963 ) ;
#58396=( NAMED_UNIT ( * ) SI_UNIT ( $, .STERADIAN. ) SOLID_ANGLE_UNIT ( ) );
#58420=ORIENTED_EDGE ( 'NONE', *, *, #31696, .F. ) ;
#58484=ORIENTED_EDGE ( 'NONE', *, *, #21190, .T. ) ;
#58504=ORIENTED_EDGE ( 'NONE', *, *, #7407, .F. ) ;
#58533=FACE_OUTER_BOUND ( 'NONE', #26191, .T. ) ;
#58560=CARTESIAN_POINT ( 'NONE',  ( 122.2516123306975402, 190.0000000000000000, -21.28179539054375624 ) ) ;
#58641=CARTESIAN_POINT ( 'NONE',  ( 427.4999999999999432, 207.5000000000000284, 0.000000000000000000 ) ) ;
#58658=EDGE_CURVE ( 'NONE', #23556, #44265, #48836, .T. ) ;
#58690=ORIENTED_EDGE ( 'NONE', *, *, #55981, .T. ) ;
#58723=CARTESIAN_POINT ( 'NONE',  ( 329.1355598199468204, 190.0000000000000000, -129.5087625010780812 ) ) ;
#58802=DIRECTION ( 'NONE',  ( 0.000000000000000000, 1.000000000000000000, -0.000000000000000000 ) ) ;
#58881=DIRECTION ( 'NONE',  ( 0.000000000000000000, 0.000000000000000000, -1.000000000000000000 ) ) ;
#58945=AXIS2_PLACEMENT_3D ( 'NONE', #44158, #13223, #1611 ) ;
#58992=DIRECTION ( 'NONE',  ( -1.000000000000000000, -0.000000000000000000, -0.000000000000000000 ) ) ;
#59004=CARTESIAN_POINT ( 'NONE',  ( -17.50000000000000000, -17.50000000000000000, 1.999999999999998224 ) ) ;
#59058=DIRECTION ( 'NONE',  ( 0.000000000000000000, 0.000000000000000000, -1.000000000000000000 ) ) ;
#59132=EDGE_LOOP ( 'NONE', ( #10125, #32341, #60946, #67429 ) ) ;
#59189=AXIS2_PLACEMENT_3D ( 'NONE', #30753, #4697, #19852 ) ;
#59258=PRODUCT_CONTEXT ( 'NONE', #35896, 'mechanical' ) ;
#59365=VERTEX_POINT ( 'NONE', #45237 ) ;
#59387=VERTEX_POINT ( 'NONE', #13245 ) ;
#59399=DIRECTION ( 'NONE',  ( -0.000000000000000000, -0.000000000000000000, 1.000000000000000000 ) ) ;
#59404=CARTESIAN_POINT ( 'NONE',  ( 122.2516123306975402, 190.0000000000000000, -91.28179539054376335 ) ) ;
#59423=AXIS2_PLACEMENT_3D ( 'NONE', #56733, #13476, #65284 ) ;
#59561=ORIENTED_EDGE ( 'NONE', *, *, #55981, .F. ) ;
#59592=CARTESIAN_POINT ( 'NONE',  ( 410.0000000000000000, 190.0000000000000000, -90.00000000000000000 ) ) ;
#59694=ADVANCED_FACE ( 'NONE', ( #66550 ), #55982, .F. ) ;
#59703=FACE_OUTER_BOUND ( 'NONE', #32540, .T. ) ;
#59773=SURFACE_STYLE_USAGE ( .BOTH. , #21132 ) ;
#59862=EDGE_CURVE ( 'NONE', #67613, #59387, #47755, .T. ) ;
#59922=ORIENTED_EDGE ( 'NONE', *, *, #55811, .F. ) ;
#59955=VECTOR ( 'NONE', #68276, 1000.000000000000000 ) ;
#59958=AXIS2_PLACEMENT_3D ( 'NONE', #16954, #17672, #49309 ) ;
#59969=VECTOR ( 'NONE', #55181, 1000.000000000000000 ) ;
#60107=CIRCLE ( 'NONE', #5079, 91.99999999999997158 ) ;
#60208=AXIS2_PLACEMENT_3D ( 'NONE', #65750, #59058, #37956 ) ;
#60400=CARTESIAN_POINT ( 'NONE',  ( 410.0000000000000000, 188.0000000000000000, -90.00000000000000000 ) ) ;
#60420=DIRECTION ( 'NONE',  ( 0.000000000000000000, 0.000000000000000000, 1.000000000000000000 ) ) ;
#60452=VERTEX_POINT ( 'NONE', #61005 ) ;
#60620=CARTESIAN_POINT ( 'NONE',  ( 450.2085304802404835, 190.0000000000000000, -219.9999999999999147 ) ) ;
#60636=VERTEX_POINT ( 'NONE', #15238 ) ;
#60687=DIRECTION ( 'NONE',  ( -0.000000000000000000, -0.000000000000000000, -1.000000000000000000 ) ) ;
#60732=DIRECTION ( 'NONE',  ( -0.000000000000000000, -1.000000000000000000, -0.000000000000000000 ) ) ;
#60735=ADVANCED_FACE ( 'NONE', ( #67179 ), #28206, .T. ) ;
#60754=ORIENTED_EDGE ( 'NONE', *, *, #34405, .F. ) ;
#60889=LINE ( 'NONE', #3206, #21517 ) ;
#60890=FACE_OUTER_BOUND ( 'NONE', #33593, .T. ) ;
#60946=ORIENTED_EDGE ( 'NONE', *, *, #11182, .F. ) ;
#61005=CARTESIAN_POINT ( 'NONE',  ( 259.2042601260359334, 188.0000000000000000, -91.27944787107685443 ) ) ;
#61083=DIRECTION ( 'NONE',  ( 0.000000000000000000, 1.000000000000000000, 0.000000000000000000 ) ) ;
#61149=CYLINDRICAL_SURFACE ( 'NONE', #29555, 299.9999999999999432 ) ;
#61158=DIRECTION ( 'NONE',  ( -0.000000000000000000, -0.000000000000000000, -1.000000000000000000 ) ) ;
#61245=EDGE_CURVE ( 'NONE', #54323, #27270, #37759, .T. ) ;
#61337=CARTESIAN_POINT ( 'NONE',  ( 329.1355598199467636, 188.0000000000000000, -129.5087625010780812 ) ) ;
#61361=CARTESIAN_POINT ( 'NONE',  ( 99.71998884745383407, 190.0000000000000000, 7.478223336038896996 ) ) ;
#61380=ADVANCED_FACE ( 'NONE', ( #29023 ), #45178, .T. ) ;
#61393=CARTESIAN_POINT ( 'NONE',  ( 99.71998884745383407, 188.0000000000000000, -91.27944787107685443 ) ) ;
#61395=CARTESIAN_POINT ( 'NONE',  ( -35.00000000000000000, -35.00000000000000000, 2.000000000000000000 ) ) ;
#61453=ADVANCED_FACE ( 'NONE', ( #30053 ), #29696, .T. ) ;
#61626=ORIENTED_EDGE ( 'NONE', *, *, #32938, .F. ) ;
#61713=DIRECTION ( 'NONE',  ( 0.000000000000000000, -1.000000000000000000, 0.000000000000000000 ) ) ;
#61723=CARTESIAN_POINT ( 'NONE',  ( 427.4999999999999432, -17.50000000000000000, 20.00000000000000000 ) ) ;
#61740=VERTEX_POINT ( 'NONE', #56008 ) ;
#61751=VERTEX_POINT ( 'NONE', #18365 ) ;
#61832=VERTEX_POINT ( 'NONE', #26414 ) ;
#61850=DIRECTION ( 'NONE',  ( -0.000000000000000000, -1.000000000000000000, -0.000000000000000000 ) ) ;
#61867=DIRECTION ( 'NONE',  ( -0.000000000000000000, -1.000000000000000000, -0.000000000000000000 ) ) ;
#61868=ORIENTED_EDGE ( 'NONE', *, *, #16598, .F. ) ;
#61881=LINE ( 'NONE', #2461, #2458 ) ;
#61928=ORIENTED_EDGE ( 'NONE', *, *, #17667, .F. ) ;
#61938=LINE ( 'NONE', #51055, #59955 ) ;
#61965=CARTESIAN_POINT ( 'NONE',  ( 450.2085304802404266, 0.000000000000000000, -250.0000000000000000 ) ) ;
#61986=VERTEX_POINT ( 'NONE', #49412 ) ;
#62055=ORIENTED_EDGE ( 'NONE', *, *, #62367, .T. ) ;
#62069=CARTESIAN_POINT ( 'NONE',  ( 47.74291447196797833, 190.0000000000000000, -75.60236247897087480 ) ) ;
#62073=VECTOR ( 'NONE', #5841, 1000.000000000000000 ) ;
#62082=EDGE_CURVE ( 'NONE', #30638, #56615, #66669, .T. ) ;
#62092=ADVANCED_FACE ( 'NONE', ( #63799 ), #31779, .F. ) ;
#62130=ORIENTED_EDGE ( 'NONE', *, *, #17667, .T. ) ;
#62164=CARTESIAN_POINT ( 'NONE',  ( 0.000000000000000000, 0.000000000000000000, 0.000000000000000000 ) ) ;
#62188=ORIENTED_EDGE ( 'NONE', *, *, #35435, .T. ) ;
#62213=DIRECTION ( 'NONE',  ( -0.9174381082928754205, 0.3978785209734126416, 0.000000000000000000 ) ) ;
#62220=VERTEX_POINT ( 'NONE', #41310 ) ;
#62255=ORIENTED_EDGE ( 'NONE', *, *, #48121, .F. ) ;
#62281=EDGE_CURVE ( 'NONE', #38976, #50879, #19327, .T. ) ;
#62288=CIRCLE ( 'NONE', #57767, 97.99999999999994316 ) ;
#62367=EDGE_CURVE ( 'NONE', #59387, #17233, #46856, .T. ) ;
#62371=CYLINDRICAL_SURFACE ( 'NONE', #16929, 299.9999999999999432 ) ;
#62411=CARTESIAN_POINT ( 'NONE',  ( 427.4999999999999432, -17.50000000000000000, 0.000000000000000000 ) ) ;
#62496=FACE_OUTER_BOUND ( 'NONE', #43135, .T. ) ;
#62503=CARTESIAN_POINT ( 'NONE',  ( 390.9212159716611836, 2.000000000000001776, 0.000000000000000000 ) ) ;
#62533=DIRECTION ( 'NONE',  ( -0.000000000000000000, 0.000000000000000000, 1.000000000000000000 ) ) ;
#62536=PLANE ( 'NONE',  #68010 ) ;
#62588=AXIS2_PLACEMENT_3D ( 'NONE', #13340, #35481, #12999 ) ;
#62633=CARTESIAN_POINT ( 'NONE',  ( 311.9732115134679020, 188.0000000000000000, -151.4173343409194672 ) ) ;
#62653=ORIENTED_EDGE ( 'NONE', *, *, #59862, .F. ) ;
#62699=ORIENTED_EDGE ( 'NONE', *, *, #5607, .F. ) ;
#62745=EDGE_CURVE ( 'NONE', #14749, #31022, #34315, .T. ) ;
#62802=DIRECTION ( 'NONE',  ( -0.000000000000000000, -1.000000000000000000, -0.000000000000000000 ) ) ;
#62814=CIRCLE ( 'NONE', #59423, 5.000000000000000888 ) ;
#62837=MECHANICAL_DESIGN_GEOMETRIC_PRESENTATION_REPRESENTATION('',(#53859),#2183);
#62840=ORIENTED_EDGE ( 'NONE', *, *, #32632, .T. ) ;
#62894=CYLINDRICAL_SURFACE ( 'NONE', #45622, 5.000000000000000888 ) ;
#62977=CARTESIAN_POINT ( 'NONE',  ( -1.148430018225554461, 500.0000000000000000, -91.64566090791306863 ) ) ;
#63013=EDGE_LOOP ( 'NONE', ( #11077, #10954, #23999, #37304 ) ) ;
#63027=DIRECTION ( 'NONE',  ( 1.000000000000000000, 0.000000000000000000, 0.000000000000000000 ) ) ;
#63031=DIRECTION ( 'NONE',  ( 0.3978782902816504485, 0.9174375763581196219, -0.001076851285082543489 ) ) ;
#63061=DIRECTION ( 'NONE',  ( 0.000000000000000000, 0.000000000000000000, -1.000000000000000000 ) ) ;
#63162=EDGE_CURVE ( 'NONE', #41559, #8207, #42600, .T. ) ;
#63200=ORIENTED_EDGE ( 'NONE', *, *, #16907, .F. ) ;
#63270=EDGE_LOOP ( 'NONE', ( #52674, #50773, #14898, #7586 ) ) ;
#63304=ORIENTED_EDGE ( 'NONE', *, *, #23457, .F. ) ;
#63403=ORIENTED_EDGE ( 'NONE', *, *, #67221, .F. ) ;
#63500=FACE_BOUND ( 'NONE', #12148, .T. ) ;
#63570=PLANE ( 'NONE',  #41960 ) ;
#63589=EDGE_CURVE ( 'NONE', #60452, #22374, #39936, .T. ) ;
#63590=ORIENTED_EDGE ( 'NONE', *, *, #44651, .T. ) ;
#63738=VECTOR ( 'NONE', #26778, 1000.000000000000000 ) ;
#63762=ORIENTED_EDGE ( 'NONE', *, *, #3064, .T. ) ;
#63772=AXIS2_PLACEMENT_3D ( 'NONE', #24785, #61713, #2633 ) ;
#63798=ORIENTED_EDGE ( 'NONE', *, *, #23136, .F. ) ;
#63799=FACE_OUTER_BOUND ( 'NONE', #11524, .T. ) ;
#63922=VECTOR ( 'NONE', #2900, 1000.000000000000000 ) ;
#63928=ORIENTED_EDGE ( 'NONE', *, *, #27948, .F. ) ;
#63953=ORIENTED_EDGE ( 'NONE', *, *, #26622, .T. ) ;
#63958=AXIS2_PLACEMENT_3D ( 'NONE', #67804, #20293, #19254 ) ;
#64017=DIRECTION ( 'NONE',  ( -0.000000000000000000, -1.000000000000000000, -0.000000000000000000 ) ) ;
#64026=EDGE_LOOP ( 'NONE', ( #66044, #3934, #55608, #40057, #52904 ) ) ;
#64165=DIRECTION ( 'NONE',  ( 0.000000000000000000, 1.000000000000000000, -0.000000000000000000 ) ) ;
#64242=EDGE_LOOP ( 'NONE', ( #62055, #67284, #63798, #26043 ) ) ;
#64377=AXIS2_PLACEMENT_3D ( 'NONE', #40377, #62533, #29824 ) ;
#64378=ORIENTED_EDGE ( 'NONE', *, *, #67508, .T. ) ;
#64486=VECTOR ( 'NONE', #21187, 1000.000000000000000 ) ;
#64592=AXIS2_PLACEMENT_3D ( 'NONE', #10410, #48037, #43109 ) ;
#64657=ORIENTED_EDGE ( 'NONE', *, *, #16765, .T. ) ;
#64671=VECTOR ( 'NONE', #42695, 1000.000000000000000 ) ;
#64683=CARTESIAN_POINT ( 'NONE',  ( 563.4809901518626702, 0.000000000000000000, 57.79371821540657095 ) ) ;
#64694=CARTESIAN_POINT ( 'NONE',  ( 311.8713128290285113, 188.0000000000000000, 346.5826552340383842 ) ) ;
#64716=ORIENTED_EDGE ( 'NONE', *, *, #11317, .F. ) ;
#64765=ADVANCED_FACE ( 'NONE', ( #56510, #41725, #29784, #51253, #24859, #24525 ), #57216, .F. ) ;
#64891=CARTESIAN_POINT ( 'NONE',  ( 410.0000000000000000, 190.0000000000000000, 0.000000000000000000 ) ) ;
#65035=ORIENTED_EDGE ( 'NONE', *, *, #56538, .T. ) ;
#65064=CARTESIAN_POINT ( 'NONE',  ( 122.2516123306975402, 190.0000000000000000, -91.28179539054376335 ) ) ;
#65110=MANIFOLD_SOLID_BREP ( 'Shell1', #36198 ) ;
#65212=DIRECTION ( 'NONE',  ( 0.000000000000000000, 0.000000000000000000, -1.000000000000000000 ) ) ;
#65264=EDGE_CURVE ( 'NONE', #60452, #52426, #42667, .T. ) ;
#65284=DIRECTION ( 'NONE',  ( 1.000000000000000000, 0.000000000000000000, 0.000000000000000000 ) ) ;
#65285=DIRECTION ( 'NONE',  ( -0.000000000000000000, -1.000000000000000000, -0.000000000000000000 ) ) ;
#65313=DIRECTION ( 'NONE',  ( -1.000000000000000000, 0.000000000000000000, 0.000000000000000000 ) ) ;
#65357=STYLED_ITEM ( 'NONE', ( #42575 ), #18036 ) ;
#65368=EDGE_CURVE ( 'NONE', #44265, #67613, #35239, .T. ) ;
#65414=CARTESIAN_POINT ( 'NONE',  ( 311.8713128290285113, 190.0000000000000000, 346.5826552340383842 ) ) ;
#65415=VERTEX_POINT ( 'NONE', #67274 ) ;
#65550=AXIS2_PLACEMENT_3D ( 'NONE', #2340, #2001, #12196 ) ;
#65611=CIRCLE ( 'NONE', #35277, 89.99999999999997158 ) ;
#65750=CARTESIAN_POINT ( 'NONE',  ( 427.4999999999999432, -17.50000000000000000, 0.000000000000000000 ) ) ;
#65759=CYLINDRICAL_SURFACE ( 'NONE', #19601, 5.000000000000004441 ) ;
#65761=ORIENTED_EDGE ( 'NONE', *, *, #56538, .F. ) ;
#65923=DIRECTION ( 'NONE',  ( 0.9268618657695262275, 0.3754025596372950191, 0.000000000000000000 ) ) ;
#65926=EDGE_LOOP ( 'NONE', ( #46027, #62653, #1353, #59561, #24899, #59922, #3473 ) ) ;
#66044=ORIENTED_EDGE ( 'NONE', *, *, #12713, .F. ) ;
#66161=EDGE_LOOP ( 'NONE', ( #64657, #43779, #27602, #40640 ) ) ;
#66200=DIRECTION ( 'NONE',  ( 0.000000000000000000, 1.000000000000000000, 0.000000000000000000 ) ) ;
#66208=EDGE_LOOP ( 'NONE', ( #68369, #61626, #43814, #12022 ) ) ;
#66228=DIRECTION ( 'NONE',  ( 0.000000000000000000, -0.9999993111447558203, 0.001173758924898823551 ) ) ;
#66248=FACE_OUTER_BOUND ( 'NONE', #49367, .T. ) ;
#66393=AXIS2_PLACEMENT_3D ( 'NONE', #35865, #51696, #2129 ) ;
#66413=ADVANCED_FACE ( 'NONE', ( #66248 ), #6779, .T. ) ;
#66468=DIRECTION ( 'NONE',  ( -0.000000000000000000, -0.000000000000000000, -1.000000000000000000 ) ) ;
#66549=VERTEX_POINT ( 'NONE', #51440 ) ;
#66550=FACE_OUTER_BOUND ( 'NONE', #57204, .T. ) ;
#66669=LINE ( 'NONE', #35339, #41242 ) ;
#66716=CARTESIAN_POINT ( 'NONE',  ( 125.2194818923508848, 188.0000000000000000, -91.27944787107685443 ) ) ;
#66760=EDGE_CURVE ( 'NONE', #17378, #14449, #67627, .T. ) ;
#66774=CIRCLE ( 'NONE', #39793, 99.99999999999994316 ) ;
#66788=EDGE_CURVE ( 'NONE', #19234, #67613, #24954, .T. ) ;
#66810=DIRECTION ( 'NONE',  ( -1.000000000000000000, 0.000000000000000000, -0.000000000000000000 ) ) ;
#66832=AXIS2_PLACEMENT_3D ( 'NONE', #50530, #44558, #8319 ) ;
#66926=DIRECTION ( 'NONE',  ( -0.000000000000000000, -1.000000000000000000, -0.000000000000000000 ) ) ;
#66967=CIRCLE ( 'NONE', #51240, 498.0000000000000000 ) ;
#67020=DIRECTION ( 'NONE',  ( -0.3754023374827052950, 0.9268613172740186590, -0.001087912492708085392 ) ) ;
#67076=AXIS2_PLACEMENT_3D ( 'NONE', #7566, #22680, #55378 ) ;
#67130=CIRCLE ( 'NONE', #52491, 5.000000000000004441 ) ;
#67167=EDGE_CURVE ( 'NONE', #30638, #37226, #33365, .T. ) ;
#67179=FACE_OUTER_BOUND ( 'NONE', #53449, .T. ) ;
#67221=EDGE_CURVE ( 'NONE', #60636, #61740, #44597, .T. ) ;
#67274=CARTESIAN_POINT ( 'NONE',  ( 422.4999999999999432, -17.50000000000000000, 0.000000000000000000 ) ) ;
#67284=ORIENTED_EDGE ( 'NONE', *, *, #29712, .F. ) ;
#67348=EDGE_LOOP ( 'NONE', ( #36618, #15021, #30422, #436 ) ) ;
#67395=CARTESIAN_POINT ( 'NONE',  ( 311.8713128290285113, 190.0000000000000000, -151.4173447659616443 ) ) ;
#67408=ORIENTED_EDGE ( 'NONE', *, *, #62082, .T. ) ;
#67427=CYLINDRICAL_SURFACE ( 'NONE', #15837, 498.0000000000000000 ) ;
#67429=ORIENTED_EDGE ( 'NONE', *, *, #49048, .T. ) ;
#67508=EDGE_CURVE ( 'NONE', #6711, #26511, #21507, .T. ) ;
#67610=LINE ( 'NONE', #57056, #41039 ) ;
#67613=VERTEX_POINT ( 'NONE', #56652 ) ;
#67627=CIRCLE ( 'NONE', #3596, 299.9999999999999432 ) ;
#67699=DIRECTION ( 'NONE',  ( 0.000000000000000000, 1.000000000000000000, -0.000000000000000000 ) ) ;
#67743=ORIENTED_EDGE ( 'NONE', *, *, #35948, .F. ) ;
#67754=SHAPE_REPRESENTATION_RELATIONSHIP ( 'NONE' , 'NONE' ,  #15003, #21404 ) ;
#67781=ORIENTED_EDGE ( 'NONE', *, *, #44934, .F. ) ;
#67804=CARTESIAN_POINT ( 'NONE',  ( 563.4809901518626702, 2.000000000000001776, 57.79371821540657095 ) ) ;
#67806=ORIENTED_EDGE ( 'NONE', *, *, #27885, .F. ) ;
#67813=DIRECTION ( 'NONE',  ( -0.000000000000000000, -1.000000000000000000, 0.000000000000000000 ) ) ;
#67855=EDGE_CURVE ( 'NONE', #56615, #11952, #5926, .T. ) ;
#67873=VECTOR ( 'NONE', #63061, 1000.000000000000000 ) ;
#67886=ORIENTED_EDGE ( 'NONE', *, *, #31290, .T. ) ;
#68010=AXIS2_PLACEMENT_3D ( 'NONE', #14349, #35804, #57256 ) ;
#68040=SURFACE_SIDE_STYLE ('',( #8943 ) ) ;
#68064=AXIS2_PLACEMENT_3D ( 'NONE', #2932, #19799, #34946 ) ;
#68163=DIRECTION ( 'NONE',  ( 1.000000000000000000, 0.000000000000000000, 0.000000000000000000 ) ) ;
#68238=LINE ( 'NONE', #58019, #27124 ) ;
#68245=EDGE_CURVE ( 'NONE', #8863, #27270, #22742, .T. ) ;
#68276=DIRECTION ( 'NONE',  ( -1.000000000000000000, 0.000000000000000000, 0.000000000000000000 ) ) ;
#68285=EDGE_CURVE ( 'NONE', #14749, #61986, #38566, .T. ) ;
#68295=ORIENTED_EDGE ( 'NONE', *, *, #55168, .T. ) ;
#68316=DIRECTION ( 'NONE',  ( -0.000000000000000000, -0.000000000000000000, -1.000000000000000000 ) ) ;
#68347=LINE ( 'NONE', #32085, #67873 ) ;
#68351=AXIS2_PLACEMENT_3D ( 'NONE', #59004, #31944, #52689 ) ;
#68369=ORIENTED_EDGE ( 'NONE', *, *, #24640, .F. ) ;
#68400=CARTESIAN_POINT ( 'NONE',  ( -22.50000000000000355, 207.5000000000000284, 1.999999999999998224 ) ) ;
#68401=LINE ( 'NONE', #62069, #54524 ) ;
#68434=DIRECTION ( 'NONE',  ( 1.000000000000000000, 0.000000000000000000, 0.000000000000000000 ) ) ;
#68445=EDGE_CURVE ( 'NONE', #60636, #34560, #4656, .T. ) ;
#68526=EDGE_CURVE ( 'NONE', #18178, #23198, #29754, .T. ) ;
#68531=EDGE_CURVE ( 'NONE', #14479, #15873, #62288, .T. ) ;
#68543=EDGE_CURVE ( 'NONE', #14449, #33323, #68347, .T. ) ;
#68609=ORIENTED_EDGE ( 'NONE', *, *, #24618, .T. ) ;
#68713=ORIENTED_EDGE ( 'NONE', *, *, #30337, .F. ) ;
#68755=VECTOR ( 'NONE', #51318, 1000.000000000000000 ) ;
#68856=VERTEX_POINT ( 'NONE', #62977 ) ;
#68964=EDGE_LOOP ( 'NONE', ( #34955, #40727, #49500, #38039 ) ) ;
#69037=ADVANCED_FACE ( 'NONE', ( #16510 ), #65759, .F. ) ;
#69040=DIRECTION ( 'NONE',  ( 0.3978782902816504485, 0.9174375763581197329, -0.001076851285082543923 ) ) ;
#69147=ORIENTED_EDGE ( 'NONE', *, *, #54944, .F. ) ;
#69192=CARTESIAN_POINT ( 'NONE',  ( 0.000000000000000000, 0.000000000000000000, 0.000000000000000000 ) ) ;
#69221=ADVANCED_FACE ( 'NONE', ( #51316, #7363 ), #2090, .F. ) ;
#69293=VECTOR ( 'NONE', #58992, 1000.000000000000000 ) ;
#69306=SURFACE_STYLE_FILL_AREA ( #16870 ) ;
#69368=CARTESIAN_POINT ( 'NONE',  ( 410.0000000000000000, 190.0000000000000000, 2.000000000000000000 ) ) ;
#69455=ORIENTED_EDGE ( 'NONE', *, *, #10170, .T. ) ;
#69456=FACE_BOUND ( 'NONE', #27876, .T. ) ;
#69468=LINE ( 'NONE', #58560, #152 ) ;
#69520=FACE_BOUND ( 'NONE', #24254, .T. ) ;
#69556=ORIENTED_EDGE ( 'NONE', *, *, #55168, .F. ) ;
#69571=FILL_AREA_STYLE_COLOUR ( '', #38382 ) ;
ENDSEC;
END-ISO-10303-21;
